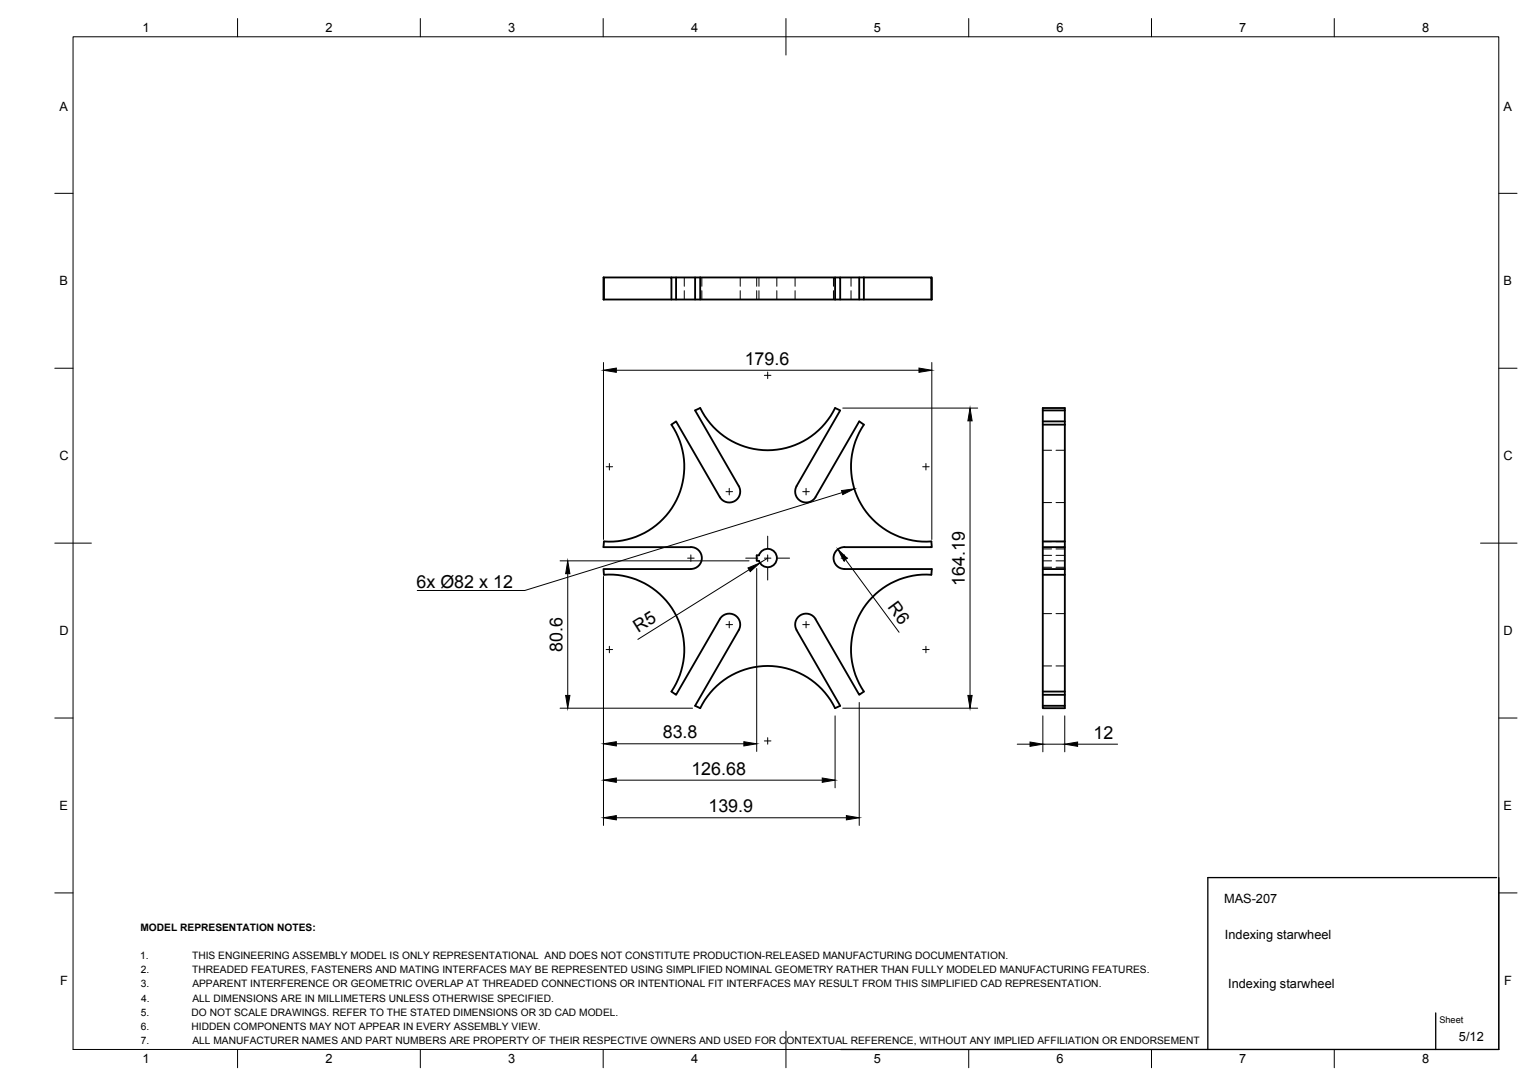
ISO-10303-21;
HEADER;
/* Generated by software containing ST-Developer
 * from STEP Tools, Inc. (www.steptools.com) 
 */

FILE_DESCRIPTION(
/* description */ ('Independent six-slot Geneva indexer. Center distance100, drive radius
50, 60degree indexing per input revolution with120degree engagement an
d240degree dwell. Native machined concave locking faces and relieved d
isk; replaceable retained drive pin; keyed output shaft. Geometry traj
ectory checks use calculated indexing positions, not a contact-dynamic
s simulation. No load or production rating assigned.'),
/* implementation_level */ '2;1');

FILE_NAME(
/* name */ 'Indexing starwheel.step',
/* time_stamp */ '2026-11-09T17:53:22-08:00',
/* author */ (''),
/* organization */ (''),
/* preprocessor_version */ 'ST-DEVELOPER v20.2',
/* originating_system */ 'Autodesk Translation Framework v15.17.0.0',
/* authorisation */ '');

FILE_SCHEMA (('AUTOMOTIVE_DESIGN { 1 0 10303 214 3 1 1 }'));
ENDSEC;

DATA;
#10=MECHANICAL_DESIGN_GEOMETRIC_PRESENTATION_REPRESENTATION('',(#103),#4149);
#81=SHAPE_REPRESENTATION_RELATIONSHIP('SRR','None',#4198,#92);
#92=ADVANCED_BREP_SHAPE_REPRESENTATION('',(#114),#4140);
#103=STYLED_ITEM('',(#4262),#114);
#114=MANIFOLD_SOLID_BREP('Body1',#2297);
#142=FACE_BOUND('',#437,.T.);
#143=FACE_BOUND('',#451,.T.);
#186=PLANE('',#2503);
#187=PLANE('',#2504);
#188=PLANE('',#2505);
#189=PLANE('',#2509);
#190=PLANE('',#2558);
#191=PLANE('',#2573);
#192=PLANE('',#2574);
#193=PLANE('',#2576);
#194=PLANE('',#2577);
#195=PLANE('',#2579);
#196=PLANE('',#2580);
#197=PLANE('',#2584);
#198=PLANE('',#2585);
#199=PLANE('',#2587);
#200=PLANE('',#2588);
#201=PLANE('',#2592);
#202=PLANE('',#2593);
#277=FACE_OUTER_BOUND('',#432,.T.);
#278=FACE_OUTER_BOUND('',#433,.T.);
#279=FACE_OUTER_BOUND('',#434,.T.);
#280=FACE_OUTER_BOUND('',#435,.T.);
#281=FACE_OUTER_BOUND('',#436,.T.);
#282=FACE_OUTER_BOUND('',#438,.T.);
#283=FACE_OUTER_BOUND('',#439,.T.);
#284=FACE_OUTER_BOUND('',#440,.T.);
#285=FACE_OUTER_BOUND('',#441,.T.);
#286=FACE_OUTER_BOUND('',#442,.T.);
#287=FACE_OUTER_BOUND('',#443,.T.);
#288=FACE_OUTER_BOUND('',#444,.T.);
#289=FACE_OUTER_BOUND('',#445,.T.);
#290=FACE_OUTER_BOUND('',#446,.T.);
#291=FACE_OUTER_BOUND('',#447,.T.);
#292=FACE_OUTER_BOUND('',#448,.T.);
#293=FACE_OUTER_BOUND('',#449,.T.);
#294=FACE_OUTER_BOUND('',#450,.T.);
#295=FACE_OUTER_BOUND('',#452,.T.);
#296=FACE_OUTER_BOUND('',#453,.T.);
#297=FACE_OUTER_BOUND('',#454,.T.);
#298=FACE_OUTER_BOUND('',#455,.T.);
#299=FACE_OUTER_BOUND('',#456,.T.);
#300=FACE_OUTER_BOUND('',#457,.T.);
#301=FACE_OUTER_BOUND('',#458,.T.);
#302=FACE_OUTER_BOUND('',#459,.T.);
#303=FACE_OUTER_BOUND('',#460,.T.);
#304=FACE_OUTER_BOUND('',#461,.T.);
#305=FACE_OUTER_BOUND('',#462,.T.);
#306=FACE_OUTER_BOUND('',#463,.T.);
#307=FACE_OUTER_BOUND('',#464,.T.);
#308=FACE_OUTER_BOUND('',#465,.T.);
#309=FACE_OUTER_BOUND('',#466,.T.);
#310=FACE_OUTER_BOUND('',#467,.T.);
#311=FACE_OUTER_BOUND('',#468,.T.);
#312=FACE_OUTER_BOUND('',#469,.T.);
#313=FACE_OUTER_BOUND('',#470,.T.);
#314=FACE_OUTER_BOUND('',#471,.T.);
#315=FACE_OUTER_BOUND('',#472,.T.);
#316=FACE_OUTER_BOUND('',#473,.T.);
#317=FACE_OUTER_BOUND('',#474,.T.);
#318=FACE_OUTER_BOUND('',#475,.T.);
#432=EDGE_LOOP('',(#1680,#1681,#1682,#1683));
#433=EDGE_LOOP('',(#1684,#1685,#1686,#1687));
#434=EDGE_LOOP('',(#1688,#1689,#1690,#1691));
#435=EDGE_LOOP('',(#1692,#1693,#1694,#1695));
#436=EDGE_LOOP('',(#1696,#1697,#1698,#1699,#1700,#1701,#1702,#1703,#1704,
#1705,#1706,#1707,#1708,#1709,#1710,#1711,#1712,#1713,#1714,#1715,#1716,
#1717,#1718,#1719,#1720,#1721,#1722,#1723,#1724,#1725,#1726,#1727,#1728,
#1729,#1730,#1731));
#437=EDGE_LOOP('',(#1732,#1733,#1734,#1735));
#438=EDGE_LOOP('',(#1736,#1737,#1738,#1739));
#439=EDGE_LOOP('',(#1740,#1741,#1742,#1743));
#440=EDGE_LOOP('',(#1744,#1745,#1746,#1747));
#441=EDGE_LOOP('',(#1748,#1749,#1750,#1751));
#442=EDGE_LOOP('',(#1752,#1753,#1754,#1755));
#443=EDGE_LOOP('',(#1756,#1757,#1758,#1759));
#444=EDGE_LOOP('',(#1760,#1761,#1762,#1763));
#445=EDGE_LOOP('',(#1764,#1765,#1766,#1767));
#446=EDGE_LOOP('',(#1768,#1769,#1770,#1771));
#447=EDGE_LOOP('',(#1772,#1773,#1774,#1775));
#448=EDGE_LOOP('',(#1776,#1777,#1778,#1779));
#449=EDGE_LOOP('',(#1780,#1781,#1782,#1783));
#450=EDGE_LOOP('',(#1784,#1785,#1786,#1787,#1788,#1789,#1790,#1791,#1792,
#1793,#1794,#1795,#1796,#1797,#1798,#1799,#1800,#1801,#1802,#1803,#1804,
#1805,#1806,#1807,#1808,#1809,#1810,#1811,#1812,#1813,#1814,#1815,#1816,
#1817,#1818,#1819));
#451=EDGE_LOOP('',(#1820,#1821,#1822,#1823));
#452=EDGE_LOOP('',(#1824,#1825,#1826,#1827));
#453=EDGE_LOOP('',(#1828,#1829,#1830,#1831));
#454=EDGE_LOOP('',(#1832,#1833,#1834,#1835));
#455=EDGE_LOOP('',(#1836,#1837,#1838,#1839));
#456=EDGE_LOOP('',(#1840,#1841,#1842,#1843));
#457=EDGE_LOOP('',(#1844,#1845,#1846,#1847));
#458=EDGE_LOOP('',(#1848,#1849,#1850,#1851));
#459=EDGE_LOOP('',(#1852,#1853,#1854,#1855));
#460=EDGE_LOOP('',(#1856,#1857,#1858,#1859));
#461=EDGE_LOOP('',(#1860,#1861,#1862,#1863));
#462=EDGE_LOOP('',(#1864,#1865,#1866,#1867));
#463=EDGE_LOOP('',(#1868,#1869,#1870,#1871));
#464=EDGE_LOOP('',(#1872,#1873,#1874,#1875));
#465=EDGE_LOOP('',(#1876,#1877,#1878,#1879));
#466=EDGE_LOOP('',(#1880,#1881,#1882,#1883));
#467=EDGE_LOOP('',(#1884,#1885,#1886,#1887));
#468=EDGE_LOOP('',(#1888,#1889,#1890,#1891));
#469=EDGE_LOOP('',(#1892,#1893,#1894,#1895));
#470=EDGE_LOOP('',(#1896,#1897,#1898,#1899));
#471=EDGE_LOOP('',(#1900,#1901,#1902,#1903));
#472=EDGE_LOOP('',(#1904,#1905,#1906,#1907));
#473=EDGE_LOOP('',(#1908,#1909,#1910,#1911));
#474=EDGE_LOOP('',(#1912,#1913,#1914,#1915));
#475=EDGE_LOOP('',(#1916,#1917,#1918,#1919));
#602=LINE('',#3655,#774);
#603=LINE('',#3657,#775);
#604=LINE('',#3659,#776);
#605=LINE('',#3660,#777);
#606=LINE('',#3664,#778);
#607=LINE('',#3666,#779);
#608=LINE('',#3668,#780);
#609=LINE('',#3669,#781);
#610=LINE('',#3671,#782);
#611=LINE('',#3672,#783);
#612=LINE('',#3683,#784);
#613=LINE('',#3687,#785);
#614=LINE('',#3695,#786);
#615=LINE('',#3699,#787);
#616=LINE('',#3707,#788);
#617=LINE('',#3711,#789);
#618=LINE('',#3719,#790);
#619=LINE('',#3723,#791);
#620=LINE('',#3731,#792);
#621=LINE('',#3735,#793);
#622=LINE('',#3743,#794);
#623=LINE('',#3747,#795);
#624=LINE('',#3751,#796);
#625=LINE('',#3753,#797);
#626=LINE('',#3757,#798);
#627=LINE('',#3759,#799);
#628=LINE('',#3763,#800);
#629=LINE('',#3765,#801);
#630=LINE('',#3769,#802);
#631=LINE('',#3771,#803);
#632=LINE('',#3775,#804);
#633=LINE('',#3777,#805);
#634=LINE('',#3781,#806);
#635=LINE('',#3784,#807);
#636=LINE('',#3787,#808);
#637=LINE('',#3792,#809);
#638=LINE('',#3795,#810);
#639=LINE('',#3799,#811);
#640=LINE('',#3803,#812);
#641=LINE('',#3807,#813);
#642=LINE('',#3811,#814);
#643=LINE('',#3815,#815);
#644=LINE('',#3818,#816);
#645=LINE('',#3822,#817);
#646=LINE('',#3825,#818);
#647=LINE('',#3829,#819);
#648=LINE('',#3832,#820);
#649=LINE('',#3836,#821);
#650=LINE('',#3839,#822);
#651=LINE('',#3843,#823);
#652=LINE('',#3848,#824);
#653=LINE('',#3851,#825);
#654=LINE('',#3853,#826);
#655=LINE('',#3855,#827);
#656=LINE('',#3857,#828);
#657=LINE('',#3859,#829);
#658=LINE('',#3862,#830);
#659=LINE('',#3863,#831);
#660=LINE('',#3865,#832);
#661=LINE('',#3868,#833);
#662=LINE('',#3869,#834);
#663=LINE('',#3871,#835);
#664=LINE('',#3876,#836);
#665=LINE('',#3877,#837);
#666=LINE('',#3879,#838);
#667=LINE('',#3882,#839);
#668=LINE('',#3883,#840);
#669=LINE('',#3885,#841);
#670=LINE('',#3890,#842);
#671=LINE('',#3892,#843);
#774=VECTOR('',#2923,10.);
#775=VECTOR('',#2924,10.);
#776=VECTOR('',#2925,10.);
#777=VECTOR('',#2926,10.);
#778=VECTOR('',#2929,10.);
#779=VECTOR('',#2930,10.);
#780=VECTOR('',#2931,10.);
#781=VECTOR('',#2932,10.);
#782=VECTOR('',#2935,10.);
#783=VECTOR('',#2936,10.);
#784=VECTOR('',#2949,10.);
#785=VECTOR('',#2952,10.);
#786=VECTOR('',#2959,10.);
#787=VECTOR('',#2962,10.);
#788=VECTOR('',#2969,10.);
#789=VECTOR('',#2972,10.);
#790=VECTOR('',#2979,10.);
#791=VECTOR('',#2982,10.);
#792=VECTOR('',#2989,10.);
#793=VECTOR('',#2992,10.);
#794=VECTOR('',#2999,10.);
#795=VECTOR('',#3002,10.);
#796=VECTOR('',#3007,10.);
#797=VECTOR('',#3008,10.);
#798=VECTOR('',#3013,10.);
#799=VECTOR('',#3014,10.);
#800=VECTOR('',#3019,10.);
#801=VECTOR('',#3020,10.);
#802=VECTOR('',#3025,10.);
#803=VECTOR('',#3026,10.);
#804=VECTOR('',#3031,10.);
#805=VECTOR('',#3032,10.);
#806=VECTOR('',#3037,10.);
#807=VECTOR('',#3040,10.);
#808=VECTOR('',#3043,10.);
#809=VECTOR('',#3050,10.);
#810=VECTOR('',#3053,10.);
#811=VECTOR('',#3058,10.);
#812=VECTOR('',#3063,10.);
#813=VECTOR('',#3068,10.);
#814=VECTOR('',#3073,10.);
#815=VECTOR('',#3076,10.);
#816=VECTOR('',#3079,10.);
#817=VECTOR('',#3082,10.);
#818=VECTOR('',#3085,10.);
#819=VECTOR('',#3088,10.);
#820=VECTOR('',#3091,10.);
#821=VECTOR('',#3094,10.);
#822=VECTOR('',#3097,10.);
#823=VECTOR('',#3100,10.);
#824=VECTOR('',#3105,10.);
#825=VECTOR('',#3108,10.);
#826=VECTOR('',#3111,10.);
#827=VECTOR('',#3114,10.);
#828=VECTOR('',#3117,10.);
#829=VECTOR('',#3120,10.);
#830=VECTOR('',#3125,10.);
#831=VECTOR('',#3126,10.);
#832=VECTOR('',#3129,10.);
#833=VECTOR('',#3134,10.);
#834=VECTOR('',#3135,10.);
#835=VECTOR('',#3138,10.);
#836=VECTOR('',#3147,10.);
#837=VECTOR('',#3148,10.);
#838=VECTOR('',#3151,10.);
#839=VECTOR('',#3156,10.);
#840=VECTOR('',#3157,10.);
#841=VECTOR('',#3160,10.);
#842=VECTOR('',#3169,10.);
#843=VECTOR('',#3172,10.);
#924=CIRCLE('',#2507,5.);
#925=CIRCLE('',#2508,5.);
#926=CIRCLE('',#2510,41.);
#927=CIRCLE('',#2511,90.);
#928=CIRCLE('',#2512,6.);
#929=CIRCLE('',#2513,90.);
#930=CIRCLE('',#2514,41.);
#931=CIRCLE('',#2515,90.);
#932=CIRCLE('',#2516,6.);
#933=CIRCLE('',#2517,90.);
#934=CIRCLE('',#2518,41.);
#935=CIRCLE('',#2519,90.);
#936=CIRCLE('',#2520,6.);
#937=CIRCLE('',#2521,90.);
#938=CIRCLE('',#2522,41.);
#939=CIRCLE('',#2523,90.);
#940=CIRCLE('',#2524,6.);
#941=CIRCLE('',#2525,90.);
#942=CIRCLE('',#2526,41.);
#943=CIRCLE('',#2527,90.);
#944=CIRCLE('',#2528,6.);
#945=CIRCLE('',#2529,90.);
#946=CIRCLE('',#2530,41.);
#947=CIRCLE('',#2531,90.);
#948=CIRCLE('',#2532,6.);
#949=CIRCLE('',#2533,90.);
#950=CIRCLE('',#2535,41.);
#951=CIRCLE('',#2537,41.);
#952=CIRCLE('',#2539,41.);
#953=CIRCLE('',#2541,41.);
#954=CIRCLE('',#2543,41.);
#955=CIRCLE('',#2545,41.);
#956=CIRCLE('',#2547,90.);
#957=CIRCLE('',#2549,90.);
#958=CIRCLE('',#2551,90.);
#959=CIRCLE('',#2553,90.);
#960=CIRCLE('',#2555,90.);
#961=CIRCLE('',#2557,90.);
#962=CIRCLE('',#2559,6.);
#963=CIRCLE('',#2560,90.);
#964=CIRCLE('',#2561,6.);
#965=CIRCLE('',#2562,90.);
#966=CIRCLE('',#2563,6.);
#967=CIRCLE('',#2564,90.);
#968=CIRCLE('',#2565,6.);
#969=CIRCLE('',#2566,90.);
#970=CIRCLE('',#2567,6.);
#971=CIRCLE('',#2568,90.);
#972=CIRCLE('',#2569,90.);
#973=CIRCLE('',#2570,6.);
#1072=VERTEX_POINT('',#3653);
#1073=VERTEX_POINT('',#3654);
#1074=VERTEX_POINT('',#3656);
#1075=VERTEX_POINT('',#3658);
#1076=VERTEX_POINT('',#3662);
#1077=VERTEX_POINT('',#3663);
#1078=VERTEX_POINT('',#3665);
#1079=VERTEX_POINT('',#3667);
#1080=VERTEX_POINT('',#3677);
#1081=VERTEX_POINT('',#3678);
#1082=VERTEX_POINT('',#3680);
#1083=VERTEX_POINT('',#3682);
#1084=VERTEX_POINT('',#3684);
#1085=VERTEX_POINT('',#3686);
#1086=VERTEX_POINT('',#3688);
#1087=VERTEX_POINT('',#3690);
#1088=VERTEX_POINT('',#3692);
#1089=VERTEX_POINT('',#3694);
#1090=VERTEX_POINT('',#3696);
#1091=VERTEX_POINT('',#3698);
#1092=VERTEX_POINT('',#3700);
#1093=VERTEX_POINT('',#3702);
#1094=VERTEX_POINT('',#3704);
#1095=VERTEX_POINT('',#3706);
#1096=VERTEX_POINT('',#3708);
#1097=VERTEX_POINT('',#3710);
#1098=VERTEX_POINT('',#3712);
#1099=VERTEX_POINT('',#3714);
#1100=VERTEX_POINT('',#3716);
#1101=VERTEX_POINT('',#3718);
#1102=VERTEX_POINT('',#3720);
#1103=VERTEX_POINT('',#3722);
#1104=VERTEX_POINT('',#3724);
#1105=VERTEX_POINT('',#3726);
#1106=VERTEX_POINT('',#3728);
#1107=VERTEX_POINT('',#3730);
#1108=VERTEX_POINT('',#3732);
#1109=VERTEX_POINT('',#3734);
#1110=VERTEX_POINT('',#3736);
#1111=VERTEX_POINT('',#3738);
#1112=VERTEX_POINT('',#3740);
#1113=VERTEX_POINT('',#3742);
#1114=VERTEX_POINT('',#3744);
#1115=VERTEX_POINT('',#3746);
#1116=VERTEX_POINT('',#3750);
#1117=VERTEX_POINT('',#3752);
#1118=VERTEX_POINT('',#3756);
#1119=VERTEX_POINT('',#3758);
#1120=VERTEX_POINT('',#3762);
#1121=VERTEX_POINT('',#3764);
#1122=VERTEX_POINT('',#3768);
#1123=VERTEX_POINT('',#3770);
#1124=VERTEX_POINT('',#3774);
#1125=VERTEX_POINT('',#3776);
#1126=VERTEX_POINT('',#3780);
#1127=VERTEX_POINT('',#3782);
#1128=VERTEX_POINT('',#3786);
#1129=VERTEX_POINT('',#3790);
#1130=VERTEX_POINT('',#3794);
#1131=VERTEX_POINT('',#3798);
#1132=VERTEX_POINT('',#3802);
#1133=VERTEX_POINT('',#3806);
#1134=VERTEX_POINT('',#3810);
#1135=VERTEX_POINT('',#3812);
#1136=VERTEX_POINT('',#3814);
#1137=VERTEX_POINT('',#3817);
#1138=VERTEX_POINT('',#3819);
#1139=VERTEX_POINT('',#3821);
#1140=VERTEX_POINT('',#3824);
#1141=VERTEX_POINT('',#3826);
#1142=VERTEX_POINT('',#3828);
#1143=VERTEX_POINT('',#3831);
#1144=VERTEX_POINT('',#3833);
#1145=VERTEX_POINT('',#3835);
#1146=VERTEX_POINT('',#3838);
#1147=VERTEX_POINT('',#3840);
#1148=VERTEX_POINT('',#3842);
#1149=VERTEX_POINT('',#3845);
#1150=VERTEX_POINT('',#3847);
#1151=VERTEX_POINT('',#3849);
#1298=EDGE_CURVE('',#1072,#1073,#602,.T.);
#1299=EDGE_CURVE('',#1074,#1072,#603,.T.);
#1300=EDGE_CURVE('',#1075,#1074,#604,.T.);
#1301=EDGE_CURVE('',#1073,#1075,#605,.T.);
#1302=EDGE_CURVE('',#1076,#1077,#606,.T.);
#1303=EDGE_CURVE('',#1078,#1076,#607,.T.);
#1304=EDGE_CURVE('',#1078,#1079,#608,.T.);
#1305=EDGE_CURVE('',#1077,#1079,#609,.T.);
#1306=EDGE_CURVE('',#1075,#1078,#610,.T.);
#1307=EDGE_CURVE('',#1079,#1074,#611,.T.);
#1308=EDGE_CURVE('',#1076,#1073,#924,.T.);
#1309=EDGE_CURVE('',#1077,#1072,#925,.T.);
#1310=EDGE_CURVE('',#1080,#1081,#926,.T.);
#1311=EDGE_CURVE('',#1081,#1082,#927,.T.);
#1312=EDGE_CURVE('',#1082,#1083,#612,.T.);
#1313=EDGE_CURVE('',#1083,#1084,#928,.T.);
#1314=EDGE_CURVE('',#1084,#1085,#613,.T.);
#1315=EDGE_CURVE('',#1085,#1086,#929,.T.);
#1316=EDGE_CURVE('',#1086,#1087,#930,.T.);
#1317=EDGE_CURVE('',#1087,#1088,#931,.T.);
#1318=EDGE_CURVE('',#1088,#1089,#614,.T.);
#1319=EDGE_CURVE('',#1089,#1090,#932,.T.);
#1320=EDGE_CURVE('',#1090,#1091,#615,.T.);
#1321=EDGE_CURVE('',#1091,#1092,#933,.T.);
#1322=EDGE_CURVE('',#1092,#1093,#934,.T.);
#1323=EDGE_CURVE('',#1093,#1094,#935,.T.);
#1324=EDGE_CURVE('',#1094,#1095,#616,.T.);
#1325=EDGE_CURVE('',#1095,#1096,#936,.T.);
#1326=EDGE_CURVE('',#1096,#1097,#617,.T.);
#1327=EDGE_CURVE('',#1097,#1098,#937,.T.);
#1328=EDGE_CURVE('',#1098,#1099,#938,.T.);
#1329=EDGE_CURVE('',#1099,#1100,#939,.T.);
#1330=EDGE_CURVE('',#1100,#1101,#618,.T.);
#1331=EDGE_CURVE('',#1101,#1102,#940,.T.);
#1332=EDGE_CURVE('',#1102,#1103,#619,.T.);
#1333=EDGE_CURVE('',#1103,#1104,#941,.T.);
#1334=EDGE_CURVE('',#1104,#1105,#942,.T.);
#1335=EDGE_CURVE('',#1105,#1106,#943,.T.);
#1336=EDGE_CURVE('',#1106,#1107,#620,.T.);
#1337=EDGE_CURVE('',#1107,#1108,#944,.T.);
#1338=EDGE_CURVE('',#1108,#1109,#621,.T.);
#1339=EDGE_CURVE('',#1109,#1110,#945,.T.);
#1340=EDGE_CURVE('',#1110,#1111,#946,.T.);
#1341=EDGE_CURVE('',#1111,#1112,#947,.T.);
#1342=EDGE_CURVE('',#1112,#1113,#622,.T.);
#1343=EDGE_CURVE('',#1113,#1114,#948,.T.);
#1344=EDGE_CURVE('',#1114,#1115,#623,.T.);
#1345=EDGE_CURVE('',#1115,#1080,#949,.T.);
#1346=EDGE_CURVE('',#1081,#1116,#624,.T.);
#1347=EDGE_CURVE('',#1117,#1080,#625,.T.);
#1348=EDGE_CURVE('',#1116,#1117,#950,.T.);
#1349=EDGE_CURVE('',#1105,#1118,#626,.T.);
#1350=EDGE_CURVE('',#1119,#1104,#627,.T.);
#1351=EDGE_CURVE('',#1118,#1119,#951,.T.);
#1352=EDGE_CURVE('',#1093,#1120,#628,.T.);
#1353=EDGE_CURVE('',#1121,#1092,#629,.T.);
#1354=EDGE_CURVE('',#1120,#1121,#952,.T.);
#1355=EDGE_CURVE('',#1099,#1122,#630,.T.);
#1356=EDGE_CURVE('',#1123,#1098,#631,.T.);
#1357=EDGE_CURVE('',#1122,#1123,#953,.T.);
#1358=EDGE_CURVE('',#1111,#1124,#632,.T.);
#1359=EDGE_CURVE('',#1125,#1110,#633,.T.);
#1360=EDGE_CURVE('',#1124,#1125,#954,.T.);
#1361=EDGE_CURVE('',#1126,#1086,#634,.T.);
#1362=EDGE_CURVE('',#1127,#1126,#955,.T.);
#1363=EDGE_CURVE('',#1087,#1127,#635,.T.);
#1364=EDGE_CURVE('',#1115,#1128,#636,.T.);
#1365=EDGE_CURVE('',#1128,#1117,#956,.T.);
#1366=EDGE_CURVE('',#1116,#1129,#957,.T.);
#1367=EDGE_CURVE('',#1129,#1082,#637,.T.);
#1368=EDGE_CURVE('',#1103,#1130,#638,.T.);
#1369=EDGE_CURVE('',#1130,#1119,#958,.T.);
#1370=EDGE_CURVE('',#1091,#1131,#639,.T.);
#1371=EDGE_CURVE('',#1131,#1121,#959,.T.);
#1372=EDGE_CURVE('',#1097,#1132,#640,.T.);
#1373=EDGE_CURVE('',#1132,#1123,#960,.T.);
#1374=EDGE_CURVE('',#1109,#1133,#641,.T.);
#1375=EDGE_CURVE('',#1133,#1125,#961,.T.);
#1376=EDGE_CURVE('',#1128,#1134,#642,.T.);
#1377=EDGE_CURVE('',#1134,#1135,#962,.T.);
#1378=EDGE_CURVE('',#1135,#1136,#643,.T.);
#1379=EDGE_CURVE('',#1124,#1136,#963,.T.);
#1380=EDGE_CURVE('',#1133,#1137,#644,.T.);
#1381=EDGE_CURVE('',#1137,#1138,#964,.T.);
#1382=EDGE_CURVE('',#1138,#1139,#645,.T.);
#1383=EDGE_CURVE('',#1118,#1139,#965,.T.);
#1384=EDGE_CURVE('',#1130,#1140,#646,.T.);
#1385=EDGE_CURVE('',#1140,#1141,#966,.T.);
#1386=EDGE_CURVE('',#1141,#1142,#647,.T.);
#1387=EDGE_CURVE('',#1122,#1142,#967,.T.);
#1388=EDGE_CURVE('',#1132,#1143,#648,.T.);
#1389=EDGE_CURVE('',#1143,#1144,#968,.T.);
#1390=EDGE_CURVE('',#1144,#1145,#649,.T.);
#1391=EDGE_CURVE('',#1120,#1145,#969,.T.);
#1392=EDGE_CURVE('',#1131,#1146,#650,.T.);
#1393=EDGE_CURVE('',#1146,#1147,#970,.T.);
#1394=EDGE_CURVE('',#1147,#1148,#651,.T.);
#1395=EDGE_CURVE('',#1127,#1148,#971,.T.);
#1396=EDGE_CURVE('',#1149,#1126,#972,.T.);
#1397=EDGE_CURVE('',#1149,#1150,#652,.T.);
#1398=EDGE_CURVE('',#1150,#1151,#973,.T.);
#1399=EDGE_CURVE('',#1151,#1129,#653,.T.);
#1400=EDGE_CURVE('',#1148,#1088,#654,.T.);
#1401=EDGE_CURVE('',#1085,#1149,#655,.T.);
#1402=EDGE_CURVE('',#1083,#1151,#656,.T.);
#1403=EDGE_CURVE('',#1084,#1150,#657,.T.);
#1404=EDGE_CURVE('',#1136,#1112,#658,.T.);
#1405=EDGE_CURVE('',#1113,#1135,#659,.T.);
#1406=EDGE_CURVE('',#1114,#1134,#660,.T.);
#1407=EDGE_CURVE('',#1139,#1106,#661,.T.);
#1408=EDGE_CURVE('',#1107,#1138,#662,.T.);
#1409=EDGE_CURVE('',#1108,#1137,#663,.T.);
#1410=EDGE_CURVE('',#1142,#1100,#664,.T.);
#1411=EDGE_CURVE('',#1101,#1141,#665,.T.);
#1412=EDGE_CURVE('',#1102,#1140,#666,.T.);
#1413=EDGE_CURVE('',#1145,#1094,#667,.T.);
#1414=EDGE_CURVE('',#1095,#1144,#668,.T.);
#1415=EDGE_CURVE('',#1096,#1143,#669,.T.);
#1416=EDGE_CURVE('',#1089,#1147,#670,.T.);
#1417=EDGE_CURVE('',#1090,#1146,#671,.T.);
#1680=ORIENTED_EDGE('',*,*,#1298,.F.);
#1681=ORIENTED_EDGE('',*,*,#1299,.F.);
#1682=ORIENTED_EDGE('',*,*,#1300,.F.);
#1683=ORIENTED_EDGE('',*,*,#1301,.F.);
#1684=ORIENTED_EDGE('',*,*,#1302,.F.);
#1685=ORIENTED_EDGE('',*,*,#1303,.F.);
#1686=ORIENTED_EDGE('',*,*,#1304,.T.);
#1687=ORIENTED_EDGE('',*,*,#1305,.F.);
#1688=ORIENTED_EDGE('',*,*,#1306,.F.);
#1689=ORIENTED_EDGE('',*,*,#1300,.T.);
#1690=ORIENTED_EDGE('',*,*,#1307,.F.);
#1691=ORIENTED_EDGE('',*,*,#1304,.F.);
#1692=ORIENTED_EDGE('',*,*,#1298,.T.);
#1693=ORIENTED_EDGE('',*,*,#1308,.F.);
#1694=ORIENTED_EDGE('',*,*,#1302,.T.);
#1695=ORIENTED_EDGE('',*,*,#1309,.T.);
#1696=ORIENTED_EDGE('',*,*,#1310,.T.);
#1697=ORIENTED_EDGE('',*,*,#1311,.T.);
#1698=ORIENTED_EDGE('',*,*,#1312,.T.);
#1699=ORIENTED_EDGE('',*,*,#1313,.T.);
#1700=ORIENTED_EDGE('',*,*,#1314,.T.);
#1701=ORIENTED_EDGE('',*,*,#1315,.T.);
#1702=ORIENTED_EDGE('',*,*,#1316,.T.);
#1703=ORIENTED_EDGE('',*,*,#1317,.T.);
#1704=ORIENTED_EDGE('',*,*,#1318,.T.);
#1705=ORIENTED_EDGE('',*,*,#1319,.T.);
#1706=ORIENTED_EDGE('',*,*,#1320,.T.);
#1707=ORIENTED_EDGE('',*,*,#1321,.T.);
#1708=ORIENTED_EDGE('',*,*,#1322,.T.);
#1709=ORIENTED_EDGE('',*,*,#1323,.T.);
#1710=ORIENTED_EDGE('',*,*,#1324,.T.);
#1711=ORIENTED_EDGE('',*,*,#1325,.T.);
#1712=ORIENTED_EDGE('',*,*,#1326,.T.);
#1713=ORIENTED_EDGE('',*,*,#1327,.T.);
#1714=ORIENTED_EDGE('',*,*,#1328,.T.);
#1715=ORIENTED_EDGE('',*,*,#1329,.T.);
#1716=ORIENTED_EDGE('',*,*,#1330,.T.);
#1717=ORIENTED_EDGE('',*,*,#1331,.T.);
#1718=ORIENTED_EDGE('',*,*,#1332,.T.);
#1719=ORIENTED_EDGE('',*,*,#1333,.T.);
#1720=ORIENTED_EDGE('',*,*,#1334,.T.);
#1721=ORIENTED_EDGE('',*,*,#1335,.T.);
#1722=ORIENTED_EDGE('',*,*,#1336,.T.);
#1723=ORIENTED_EDGE('',*,*,#1337,.T.);
#1724=ORIENTED_EDGE('',*,*,#1338,.T.);
#1725=ORIENTED_EDGE('',*,*,#1339,.T.);
#1726=ORIENTED_EDGE('',*,*,#1340,.T.);
#1727=ORIENTED_EDGE('',*,*,#1341,.T.);
#1728=ORIENTED_EDGE('',*,*,#1342,.T.);
#1729=ORIENTED_EDGE('',*,*,#1343,.T.);
#1730=ORIENTED_EDGE('',*,*,#1344,.T.);
#1731=ORIENTED_EDGE('',*,*,#1345,.T.);
#1732=ORIENTED_EDGE('',*,*,#1301,.T.);
#1733=ORIENTED_EDGE('',*,*,#1306,.T.);
#1734=ORIENTED_EDGE('',*,*,#1303,.T.);
#1735=ORIENTED_EDGE('',*,*,#1308,.T.);
#1736=ORIENTED_EDGE('',*,*,#1346,.F.);
#1737=ORIENTED_EDGE('',*,*,#1310,.F.);
#1738=ORIENTED_EDGE('',*,*,#1347,.F.);
#1739=ORIENTED_EDGE('',*,*,#1348,.F.);
#1740=ORIENTED_EDGE('',*,*,#1349,.F.);
#1741=ORIENTED_EDGE('',*,*,#1334,.F.);
#1742=ORIENTED_EDGE('',*,*,#1350,.F.);
#1743=ORIENTED_EDGE('',*,*,#1351,.F.);
#1744=ORIENTED_EDGE('',*,*,#1352,.F.);
#1745=ORIENTED_EDGE('',*,*,#1322,.F.);
#1746=ORIENTED_EDGE('',*,*,#1353,.F.);
#1747=ORIENTED_EDGE('',*,*,#1354,.F.);
#1748=ORIENTED_EDGE('',*,*,#1355,.F.);
#1749=ORIENTED_EDGE('',*,*,#1328,.F.);
#1750=ORIENTED_EDGE('',*,*,#1356,.F.);
#1751=ORIENTED_EDGE('',*,*,#1357,.F.);
#1752=ORIENTED_EDGE('',*,*,#1358,.F.);
#1753=ORIENTED_EDGE('',*,*,#1340,.F.);
#1754=ORIENTED_EDGE('',*,*,#1359,.F.);
#1755=ORIENTED_EDGE('',*,*,#1360,.F.);
#1756=ORIENTED_EDGE('',*,*,#1361,.F.);
#1757=ORIENTED_EDGE('',*,*,#1362,.F.);
#1758=ORIENTED_EDGE('',*,*,#1363,.F.);
#1759=ORIENTED_EDGE('',*,*,#1316,.F.);
#1760=ORIENTED_EDGE('',*,*,#1347,.T.);
#1761=ORIENTED_EDGE('',*,*,#1345,.F.);
#1762=ORIENTED_EDGE('',*,*,#1364,.T.);
#1763=ORIENTED_EDGE('',*,*,#1365,.T.);
#1764=ORIENTED_EDGE('',*,*,#1346,.T.);
#1765=ORIENTED_EDGE('',*,*,#1366,.T.);
#1766=ORIENTED_EDGE('',*,*,#1367,.T.);
#1767=ORIENTED_EDGE('',*,*,#1311,.F.);
#1768=ORIENTED_EDGE('',*,*,#1350,.T.);
#1769=ORIENTED_EDGE('',*,*,#1333,.F.);
#1770=ORIENTED_EDGE('',*,*,#1368,.T.);
#1771=ORIENTED_EDGE('',*,*,#1369,.T.);
#1772=ORIENTED_EDGE('',*,*,#1353,.T.);
#1773=ORIENTED_EDGE('',*,*,#1321,.F.);
#1774=ORIENTED_EDGE('',*,*,#1370,.T.);
#1775=ORIENTED_EDGE('',*,*,#1371,.T.);
#1776=ORIENTED_EDGE('',*,*,#1356,.T.);
#1777=ORIENTED_EDGE('',*,*,#1327,.F.);
#1778=ORIENTED_EDGE('',*,*,#1372,.T.);
#1779=ORIENTED_EDGE('',*,*,#1373,.T.);
#1780=ORIENTED_EDGE('',*,*,#1359,.T.);
#1781=ORIENTED_EDGE('',*,*,#1339,.F.);
#1782=ORIENTED_EDGE('',*,*,#1374,.T.);
#1783=ORIENTED_EDGE('',*,*,#1375,.T.);
#1784=ORIENTED_EDGE('',*,*,#1348,.T.);
#1785=ORIENTED_EDGE('',*,*,#1365,.F.);
#1786=ORIENTED_EDGE('',*,*,#1376,.T.);
#1787=ORIENTED_EDGE('',*,*,#1377,.T.);
#1788=ORIENTED_EDGE('',*,*,#1378,.T.);
#1789=ORIENTED_EDGE('',*,*,#1379,.F.);
#1790=ORIENTED_EDGE('',*,*,#1360,.T.);
#1791=ORIENTED_EDGE('',*,*,#1375,.F.);
#1792=ORIENTED_EDGE('',*,*,#1380,.T.);
#1793=ORIENTED_EDGE('',*,*,#1381,.T.);
#1794=ORIENTED_EDGE('',*,*,#1382,.T.);
#1795=ORIENTED_EDGE('',*,*,#1383,.F.);
#1796=ORIENTED_EDGE('',*,*,#1351,.T.);
#1797=ORIENTED_EDGE('',*,*,#1369,.F.);
#1798=ORIENTED_EDGE('',*,*,#1384,.T.);
#1799=ORIENTED_EDGE('',*,*,#1385,.T.);
#1800=ORIENTED_EDGE('',*,*,#1386,.T.);
#1801=ORIENTED_EDGE('',*,*,#1387,.F.);
#1802=ORIENTED_EDGE('',*,*,#1357,.T.);
#1803=ORIENTED_EDGE('',*,*,#1373,.F.);
#1804=ORIENTED_EDGE('',*,*,#1388,.T.);
#1805=ORIENTED_EDGE('',*,*,#1389,.T.);
#1806=ORIENTED_EDGE('',*,*,#1390,.T.);
#1807=ORIENTED_EDGE('',*,*,#1391,.F.);
#1808=ORIENTED_EDGE('',*,*,#1354,.T.);
#1809=ORIENTED_EDGE('',*,*,#1371,.F.);
#1810=ORIENTED_EDGE('',*,*,#1392,.T.);
#1811=ORIENTED_EDGE('',*,*,#1393,.T.);
#1812=ORIENTED_EDGE('',*,*,#1394,.T.);
#1813=ORIENTED_EDGE('',*,*,#1395,.F.);
#1814=ORIENTED_EDGE('',*,*,#1362,.T.);
#1815=ORIENTED_EDGE('',*,*,#1396,.F.);
#1816=ORIENTED_EDGE('',*,*,#1397,.T.);
#1817=ORIENTED_EDGE('',*,*,#1398,.T.);
#1818=ORIENTED_EDGE('',*,*,#1399,.T.);
#1819=ORIENTED_EDGE('',*,*,#1366,.F.);
#1820=ORIENTED_EDGE('',*,*,#1299,.T.);
#1821=ORIENTED_EDGE('',*,*,#1309,.F.);
#1822=ORIENTED_EDGE('',*,*,#1305,.T.);
#1823=ORIENTED_EDGE('',*,*,#1307,.T.);
#1824=ORIENTED_EDGE('',*,*,#1363,.T.);
#1825=ORIENTED_EDGE('',*,*,#1395,.T.);
#1826=ORIENTED_EDGE('',*,*,#1400,.T.);
#1827=ORIENTED_EDGE('',*,*,#1317,.F.);
#1828=ORIENTED_EDGE('',*,*,#1361,.T.);
#1829=ORIENTED_EDGE('',*,*,#1315,.F.);
#1830=ORIENTED_EDGE('',*,*,#1401,.T.);
#1831=ORIENTED_EDGE('',*,*,#1396,.T.);
#1832=ORIENTED_EDGE('',*,*,#1367,.F.);
#1833=ORIENTED_EDGE('',*,*,#1399,.F.);
#1834=ORIENTED_EDGE('',*,*,#1402,.F.);
#1835=ORIENTED_EDGE('',*,*,#1312,.F.);
#1836=ORIENTED_EDGE('',*,*,#1401,.F.);
#1837=ORIENTED_EDGE('',*,*,#1314,.F.);
#1838=ORIENTED_EDGE('',*,*,#1403,.T.);
#1839=ORIENTED_EDGE('',*,*,#1397,.F.);
#1840=ORIENTED_EDGE('',*,*,#1313,.F.);
#1841=ORIENTED_EDGE('',*,*,#1402,.T.);
#1842=ORIENTED_EDGE('',*,*,#1398,.F.);
#1843=ORIENTED_EDGE('',*,*,#1403,.F.);
#1844=ORIENTED_EDGE('',*,*,#1404,.F.);
#1845=ORIENTED_EDGE('',*,*,#1378,.F.);
#1846=ORIENTED_EDGE('',*,*,#1405,.F.);
#1847=ORIENTED_EDGE('',*,*,#1342,.F.);
#1848=ORIENTED_EDGE('',*,*,#1364,.F.);
#1849=ORIENTED_EDGE('',*,*,#1344,.F.);
#1850=ORIENTED_EDGE('',*,*,#1406,.T.);
#1851=ORIENTED_EDGE('',*,*,#1376,.F.);
#1852=ORIENTED_EDGE('',*,*,#1343,.F.);
#1853=ORIENTED_EDGE('',*,*,#1405,.T.);
#1854=ORIENTED_EDGE('',*,*,#1377,.F.);
#1855=ORIENTED_EDGE('',*,*,#1406,.F.);
#1856=ORIENTED_EDGE('',*,*,#1407,.F.);
#1857=ORIENTED_EDGE('',*,*,#1382,.F.);
#1858=ORIENTED_EDGE('',*,*,#1408,.F.);
#1859=ORIENTED_EDGE('',*,*,#1336,.F.);
#1860=ORIENTED_EDGE('',*,*,#1374,.F.);
#1861=ORIENTED_EDGE('',*,*,#1338,.F.);
#1862=ORIENTED_EDGE('',*,*,#1409,.T.);
#1863=ORIENTED_EDGE('',*,*,#1380,.F.);
#1864=ORIENTED_EDGE('',*,*,#1337,.F.);
#1865=ORIENTED_EDGE('',*,*,#1408,.T.);
#1866=ORIENTED_EDGE('',*,*,#1381,.F.);
#1867=ORIENTED_EDGE('',*,*,#1409,.F.);
#1868=ORIENTED_EDGE('',*,*,#1358,.T.);
#1869=ORIENTED_EDGE('',*,*,#1379,.T.);
#1870=ORIENTED_EDGE('',*,*,#1404,.T.);
#1871=ORIENTED_EDGE('',*,*,#1341,.F.);
#1872=ORIENTED_EDGE('',*,*,#1349,.T.);
#1873=ORIENTED_EDGE('',*,*,#1383,.T.);
#1874=ORIENTED_EDGE('',*,*,#1407,.T.);
#1875=ORIENTED_EDGE('',*,*,#1335,.F.);
#1876=ORIENTED_EDGE('',*,*,#1410,.F.);
#1877=ORIENTED_EDGE('',*,*,#1386,.F.);
#1878=ORIENTED_EDGE('',*,*,#1411,.F.);
#1879=ORIENTED_EDGE('',*,*,#1330,.F.);
#1880=ORIENTED_EDGE('',*,*,#1368,.F.);
#1881=ORIENTED_EDGE('',*,*,#1332,.F.);
#1882=ORIENTED_EDGE('',*,*,#1412,.T.);
#1883=ORIENTED_EDGE('',*,*,#1384,.F.);
#1884=ORIENTED_EDGE('',*,*,#1331,.F.);
#1885=ORIENTED_EDGE('',*,*,#1411,.T.);
#1886=ORIENTED_EDGE('',*,*,#1385,.F.);
#1887=ORIENTED_EDGE('',*,*,#1412,.F.);
#1888=ORIENTED_EDGE('',*,*,#1413,.F.);
#1889=ORIENTED_EDGE('',*,*,#1390,.F.);
#1890=ORIENTED_EDGE('',*,*,#1414,.F.);
#1891=ORIENTED_EDGE('',*,*,#1324,.F.);
#1892=ORIENTED_EDGE('',*,*,#1372,.F.);
#1893=ORIENTED_EDGE('',*,*,#1326,.F.);
#1894=ORIENTED_EDGE('',*,*,#1415,.T.);
#1895=ORIENTED_EDGE('',*,*,#1388,.F.);
#1896=ORIENTED_EDGE('',*,*,#1325,.F.);
#1897=ORIENTED_EDGE('',*,*,#1414,.T.);
#1898=ORIENTED_EDGE('',*,*,#1389,.F.);
#1899=ORIENTED_EDGE('',*,*,#1415,.F.);
#1900=ORIENTED_EDGE('',*,*,#1355,.T.);
#1901=ORIENTED_EDGE('',*,*,#1387,.T.);
#1902=ORIENTED_EDGE('',*,*,#1410,.T.);
#1903=ORIENTED_EDGE('',*,*,#1329,.F.);
#1904=ORIENTED_EDGE('',*,*,#1352,.T.);
#1905=ORIENTED_EDGE('',*,*,#1391,.T.);
#1906=ORIENTED_EDGE('',*,*,#1413,.T.);
#1907=ORIENTED_EDGE('',*,*,#1323,.F.);
#1908=ORIENTED_EDGE('',*,*,#1400,.F.);
#1909=ORIENTED_EDGE('',*,*,#1394,.F.);
#1910=ORIENTED_EDGE('',*,*,#1416,.F.);
#1911=ORIENTED_EDGE('',*,*,#1318,.F.);
#1912=ORIENTED_EDGE('',*,*,#1370,.F.);
#1913=ORIENTED_EDGE('',*,*,#1320,.F.);
#1914=ORIENTED_EDGE('',*,*,#1417,.T.);
#1915=ORIENTED_EDGE('',*,*,#1392,.F.);
#1916=ORIENTED_EDGE('',*,*,#1319,.F.);
#1917=ORIENTED_EDGE('',*,*,#1416,.T.);
#1918=ORIENTED_EDGE('',*,*,#1393,.F.);
#1919=ORIENTED_EDGE('',*,*,#1417,.F.);
#2114=CYLINDRICAL_SURFACE('',#2506,5.);
#2115=CYLINDRICAL_SURFACE('',#2534,41.);
#2116=CYLINDRICAL_SURFACE('',#2536,41.);
#2117=CYLINDRICAL_SURFACE('',#2538,41.);
#2118=CYLINDRICAL_SURFACE('',#2540,41.);
#2119=CYLINDRICAL_SURFACE('',#2542,41.);
#2120=CYLINDRICAL_SURFACE('',#2544,41.);
#2121=CYLINDRICAL_SURFACE('',#2546,90.);
#2122=CYLINDRICAL_SURFACE('',#2548,90.);
#2123=CYLINDRICAL_SURFACE('',#2550,90.);
#2124=CYLINDRICAL_SURFACE('',#2552,90.);
#2125=CYLINDRICAL_SURFACE('',#2554,90.);
#2126=CYLINDRICAL_SURFACE('',#2556,90.);
#2127=CYLINDRICAL_SURFACE('',#2571,90.);
#2128=CYLINDRICAL_SURFACE('',#2572,90.);
#2129=CYLINDRICAL_SURFACE('',#2575,6.);
#2130=CYLINDRICAL_SURFACE('',#2578,6.);
#2131=CYLINDRICAL_SURFACE('',#2581,6.);
#2132=CYLINDRICAL_SURFACE('',#2582,90.);
#2133=CYLINDRICAL_SURFACE('',#2583,90.);
#2134=CYLINDRICAL_SURFACE('',#2586,6.);
#2135=CYLINDRICAL_SURFACE('',#2589,6.);
#2136=CYLINDRICAL_SURFACE('',#2590,90.);
#2137=CYLINDRICAL_SURFACE('',#2591,90.);
#2138=CYLINDRICAL_SURFACE('',#2594,6.);
#2198=ADVANCED_FACE('',(#277),#186,.F.);
#2199=ADVANCED_FACE('',(#278),#187,.F.);
#2200=ADVANCED_FACE('',(#279),#188,.F.);
#2201=ADVANCED_FACE('',(#280),#2114,.F.);
#2202=ADVANCED_FACE('',(#281,#142),#189,.T.);
#2203=ADVANCED_FACE('',(#282),#2115,.F.);
#2204=ADVANCED_FACE('',(#283),#2116,.F.);
#2205=ADVANCED_FACE('',(#284),#2117,.F.);
#2206=ADVANCED_FACE('',(#285),#2118,.F.);
#2207=ADVANCED_FACE('',(#286),#2119,.F.);
#2208=ADVANCED_FACE('',(#287),#2120,.F.);
#2209=ADVANCED_FACE('',(#288),#2121,.T.);
#2210=ADVANCED_FACE('',(#289),#2122,.T.);
#2211=ADVANCED_FACE('',(#290),#2123,.T.);
#2212=ADVANCED_FACE('',(#291),#2124,.T.);
#2213=ADVANCED_FACE('',(#292),#2125,.T.);
#2214=ADVANCED_FACE('',(#293),#2126,.T.);
#2215=ADVANCED_FACE('',(#294,#143),#190,.F.);
#2216=ADVANCED_FACE('',(#295),#2127,.T.);
#2217=ADVANCED_FACE('',(#296),#2128,.T.);
#2218=ADVANCED_FACE('',(#297),#191,.F.);
#2219=ADVANCED_FACE('',(#298),#192,.F.);
#2220=ADVANCED_FACE('',(#299),#2129,.F.);
#2221=ADVANCED_FACE('',(#300),#193,.F.);
#2222=ADVANCED_FACE('',(#301),#194,.F.);
#2223=ADVANCED_FACE('',(#302),#2130,.F.);
#2224=ADVANCED_FACE('',(#303),#195,.F.);
#2225=ADVANCED_FACE('',(#304),#196,.F.);
#2226=ADVANCED_FACE('',(#305),#2131,.F.);
#2227=ADVANCED_FACE('',(#306),#2132,.T.);
#2228=ADVANCED_FACE('',(#307),#2133,.T.);
#2229=ADVANCED_FACE('',(#308),#197,.F.);
#2230=ADVANCED_FACE('',(#309),#198,.F.);
#2231=ADVANCED_FACE('',(#310),#2134,.F.);
#2232=ADVANCED_FACE('',(#311),#199,.F.);
#2233=ADVANCED_FACE('',(#312),#200,.F.);
#2234=ADVANCED_FACE('',(#313),#2135,.F.);
#2235=ADVANCED_FACE('',(#314),#2136,.T.);
#2236=ADVANCED_FACE('',(#315),#2137,.T.);
#2237=ADVANCED_FACE('',(#316),#201,.F.);
#2238=ADVANCED_FACE('',(#317),#202,.F.);
#2239=ADVANCED_FACE('',(#318),#2138,.F.);
#2297=CLOSED_SHELL('',(#2198,#2199,#2200,#2201,#2202,#2203,#2204,#2205,
#2206,#2207,#2208,#2209,#2210,#2211,#2212,#2213,#2214,#2215,#2216,#2217,
#2218,#2219,#2220,#2221,#2222,#2223,#2224,#2225,#2226,#2227,#2228,#2229,
#2230,#2231,#2232,#2233,#2234,#2235,#2236,#2237,#2238,#2239));
#2502=AXIS2_PLACEMENT_3D('',#3651,#2919,#2920);
#2503=AXIS2_PLACEMENT_3D('',#3652,#2921,#2922);
#2504=AXIS2_PLACEMENT_3D('',#3661,#2927,#2928);
#2505=AXIS2_PLACEMENT_3D('',#3670,#2933,#2934);
#2506=AXIS2_PLACEMENT_3D('',#3673,#2937,#2938);
#2507=AXIS2_PLACEMENT_3D('',#3674,#2939,#2940);
#2508=AXIS2_PLACEMENT_3D('',#3675,#2941,#2942);
#2509=AXIS2_PLACEMENT_3D('',#3676,#2943,#2944);
#2510=AXIS2_PLACEMENT_3D('',#3679,#2945,#2946);
#2511=AXIS2_PLACEMENT_3D('',#3681,#2947,#2948);
#2512=AXIS2_PLACEMENT_3D('',#3685,#2950,#2951);
#2513=AXIS2_PLACEMENT_3D('',#3689,#2953,#2954);
#2514=AXIS2_PLACEMENT_3D('',#3691,#2955,#2956);
#2515=AXIS2_PLACEMENT_3D('',#3693,#2957,#2958);
#2516=AXIS2_PLACEMENT_3D('',#3697,#2960,#2961);
#2517=AXIS2_PLACEMENT_3D('',#3701,#2963,#2964);
#2518=AXIS2_PLACEMENT_3D('',#3703,#2965,#2966);
#2519=AXIS2_PLACEMENT_3D('',#3705,#2967,#2968);
#2520=AXIS2_PLACEMENT_3D('',#3709,#2970,#2971);
#2521=AXIS2_PLACEMENT_3D('',#3713,#2973,#2974);
#2522=AXIS2_PLACEMENT_3D('',#3715,#2975,#2976);
#2523=AXIS2_PLACEMENT_3D('',#3717,#2977,#2978);
#2524=AXIS2_PLACEMENT_3D('',#3721,#2980,#2981);
#2525=AXIS2_PLACEMENT_3D('',#3725,#2983,#2984);
#2526=AXIS2_PLACEMENT_3D('',#3727,#2985,#2986);
#2527=AXIS2_PLACEMENT_3D('',#3729,#2987,#2988);
#2528=AXIS2_PLACEMENT_3D('',#3733,#2990,#2991);
#2529=AXIS2_PLACEMENT_3D('',#3737,#2993,#2994);
#2530=AXIS2_PLACEMENT_3D('',#3739,#2995,#2996);
#2531=AXIS2_PLACEMENT_3D('',#3741,#2997,#2998);
#2532=AXIS2_PLACEMENT_3D('',#3745,#3000,#3001);
#2533=AXIS2_PLACEMENT_3D('',#3748,#3003,#3004);
#2534=AXIS2_PLACEMENT_3D('',#3749,#3005,#3006);
#2535=AXIS2_PLACEMENT_3D('',#3754,#3009,#3010);
#2536=AXIS2_PLACEMENT_3D('',#3755,#3011,#3012);
#2537=AXIS2_PLACEMENT_3D('',#3760,#3015,#3016);
#2538=AXIS2_PLACEMENT_3D('',#3761,#3017,#3018);
#2539=AXIS2_PLACEMENT_3D('',#3766,#3021,#3022);
#2540=AXIS2_PLACEMENT_3D('',#3767,#3023,#3024);
#2541=AXIS2_PLACEMENT_3D('',#3772,#3027,#3028);
#2542=AXIS2_PLACEMENT_3D('',#3773,#3029,#3030);
#2543=AXIS2_PLACEMENT_3D('',#3778,#3033,#3034);
#2544=AXIS2_PLACEMENT_3D('',#3779,#3035,#3036);
#2545=AXIS2_PLACEMENT_3D('',#3783,#3038,#3039);
#2546=AXIS2_PLACEMENT_3D('',#3785,#3041,#3042);
#2547=AXIS2_PLACEMENT_3D('',#3788,#3044,#3045);
#2548=AXIS2_PLACEMENT_3D('',#3789,#3046,#3047);
#2549=AXIS2_PLACEMENT_3D('',#3791,#3048,#3049);
#2550=AXIS2_PLACEMENT_3D('',#3793,#3051,#3052);
#2551=AXIS2_PLACEMENT_3D('',#3796,#3054,#3055);
#2552=AXIS2_PLACEMENT_3D('',#3797,#3056,#3057);
#2553=AXIS2_PLACEMENT_3D('',#3800,#3059,#3060);
#2554=AXIS2_PLACEMENT_3D('',#3801,#3061,#3062);
#2555=AXIS2_PLACEMENT_3D('',#3804,#3064,#3065);
#2556=AXIS2_PLACEMENT_3D('',#3805,#3066,#3067);
#2557=AXIS2_PLACEMENT_3D('',#3808,#3069,#3070);
#2558=AXIS2_PLACEMENT_3D('',#3809,#3071,#3072);
#2559=AXIS2_PLACEMENT_3D('',#3813,#3074,#3075);
#2560=AXIS2_PLACEMENT_3D('',#3816,#3077,#3078);
#2561=AXIS2_PLACEMENT_3D('',#3820,#3080,#3081);
#2562=AXIS2_PLACEMENT_3D('',#3823,#3083,#3084);
#2563=AXIS2_PLACEMENT_3D('',#3827,#3086,#3087);
#2564=AXIS2_PLACEMENT_3D('',#3830,#3089,#3090);
#2565=AXIS2_PLACEMENT_3D('',#3834,#3092,#3093);
#2566=AXIS2_PLACEMENT_3D('',#3837,#3095,#3096);
#2567=AXIS2_PLACEMENT_3D('',#3841,#3098,#3099);
#2568=AXIS2_PLACEMENT_3D('',#3844,#3101,#3102);
#2569=AXIS2_PLACEMENT_3D('',#3846,#3103,#3104);
#2570=AXIS2_PLACEMENT_3D('',#3850,#3106,#3107);
#2571=AXIS2_PLACEMENT_3D('',#3852,#3109,#3110);
#2572=AXIS2_PLACEMENT_3D('',#3854,#3112,#3113);
#2573=AXIS2_PLACEMENT_3D('',#3856,#3115,#3116);
#2574=AXIS2_PLACEMENT_3D('',#3858,#3118,#3119);
#2575=AXIS2_PLACEMENT_3D('',#3860,#3121,#3122);
#2576=AXIS2_PLACEMENT_3D('',#3861,#3123,#3124);
#2577=AXIS2_PLACEMENT_3D('',#3864,#3127,#3128);
#2578=AXIS2_PLACEMENT_3D('',#3866,#3130,#3131);
#2579=AXIS2_PLACEMENT_3D('',#3867,#3132,#3133);
#2580=AXIS2_PLACEMENT_3D('',#3870,#3136,#3137);
#2581=AXIS2_PLACEMENT_3D('',#3872,#3139,#3140);
#2582=AXIS2_PLACEMENT_3D('',#3873,#3141,#3142);
#2583=AXIS2_PLACEMENT_3D('',#3874,#3143,#3144);
#2584=AXIS2_PLACEMENT_3D('',#3875,#3145,#3146);
#2585=AXIS2_PLACEMENT_3D('',#3878,#3149,#3150);
#2586=AXIS2_PLACEMENT_3D('',#3880,#3152,#3153);
#2587=AXIS2_PLACEMENT_3D('',#3881,#3154,#3155);
#2588=AXIS2_PLACEMENT_3D('',#3884,#3158,#3159);
#2589=AXIS2_PLACEMENT_3D('',#3886,#3161,#3162);
#2590=AXIS2_PLACEMENT_3D('',#3887,#3163,#3164);
#2591=AXIS2_PLACEMENT_3D('',#3888,#3165,#3166);
#2592=AXIS2_PLACEMENT_3D('',#3889,#3167,#3168);
#2593=AXIS2_PLACEMENT_3D('',#3891,#3170,#3171);
#2594=AXIS2_PLACEMENT_3D('',#3893,#3173,#3174);
#2919=DIRECTION('axis',(0.,0.,1.));
#2920=DIRECTION('refdir',(1.,0.,0.));
#2921=DIRECTION('center_axis',(0.,1.,0.));
#2922=DIRECTION('ref_axis',(1.,0.,0.));
#2923=DIRECTION('',(0.,0.,1.));
#2924=DIRECTION('',(-1.,0.,0.));
#2925=DIRECTION('',(0.,0.,-1.));
#2926=DIRECTION('',(1.,0.,0.));
#2927=DIRECTION('center_axis',(0.,-1.,0.));
#2928=DIRECTION('ref_axis',(-1.,0.,0.));
#2929=DIRECTION('',(0.,0.,-1.));
#2930=DIRECTION('',(-1.,0.,0.));
#2931=DIRECTION('',(0.,0.,-1.));
#2932=DIRECTION('',(1.,0.,0.));
#2933=DIRECTION('center_axis',(1.,0.,0.));
#2934=DIRECTION('ref_axis',(0.,-1.,0.));
#2935=DIRECTION('',(0.,-1.,0.));
#2936=DIRECTION('',(0.,1.,0.));
#2937=DIRECTION('center_axis',(0.,0.,1.));
#2938=DIRECTION('ref_axis',(-1.,1.22464679914735E-16,0.));
#2939=DIRECTION('center_axis',(0.,0.,-1.));
#2940=DIRECTION('ref_axis',(1.,0.,0.));
#2941=DIRECTION('center_axis',(0.,0.,-1.));
#2942=DIRECTION('ref_axis',(1.,0.,0.));
#2943=DIRECTION('center_axis',(0.,0.,1.));
#2944=DIRECTION('ref_axis',(1.,0.,0.));
#2945=DIRECTION('center_axis',(0.,0.,-1.));
#2946=DIRECTION('ref_axis',(1.,0.,0.));
#2947=DIRECTION('center_axis',(0.,0.,1.));
#2948=DIRECTION('ref_axis',(1.,0.,0.));
#2949=DIRECTION('',(-0.5,0.866025403784439,0.));
#2950=DIRECTION('center_axis',(0.,0.,-1.));
#2951=DIRECTION('ref_axis',(0.866025403784439,0.5,0.));
#2952=DIRECTION('',(0.5,-0.866025403784439,0.));
#2953=DIRECTION('center_axis',(0.,0.,1.));
#2954=DIRECTION('ref_axis',(1.,0.,0.));
#2955=DIRECTION('center_axis',(0.,0.,-1.));
#2956=DIRECTION('ref_axis',(1.,0.,0.));
#2957=DIRECTION('center_axis',(0.,0.,1.));
#2958=DIRECTION('ref_axis',(1.,0.,0.));
#2959=DIRECTION('',(-1.,0.,0.));
#2960=DIRECTION('center_axis',(0.,0.,-1.));
#2961=DIRECTION('ref_axis',(0.,1.,0.));
#2962=DIRECTION('',(1.,0.,0.));
#2963=DIRECTION('center_axis',(0.,0.,1.));
#2964=DIRECTION('ref_axis',(1.,0.,0.));
#2965=DIRECTION('center_axis',(0.,0.,-1.));
#2966=DIRECTION('ref_axis',(1.,0.,0.));
#2967=DIRECTION('center_axis',(0.,0.,1.));
#2968=DIRECTION('ref_axis',(1.,0.,0.));
#2969=DIRECTION('',(-0.5,-0.866025403784439,0.));
#2970=DIRECTION('center_axis',(0.,0.,-1.));
#2971=DIRECTION('ref_axis',(-0.866025403784439,0.5,0.));
#2972=DIRECTION('',(0.5,0.866025403784439,0.));
#2973=DIRECTION('center_axis',(0.,0.,1.));
#2974=DIRECTION('ref_axis',(1.,0.,0.));
#2975=DIRECTION('center_axis',(0.,0.,-1.));
#2976=DIRECTION('ref_axis',(1.,0.,0.));
#2977=DIRECTION('center_axis',(0.,0.,1.));
#2978=DIRECTION('ref_axis',(1.,0.,0.));
#2979=DIRECTION('',(0.5,-0.866025403784439,0.));
#2980=DIRECTION('center_axis',(0.,0.,-1.));
#2981=DIRECTION('ref_axis',(-0.866025403784439,-0.5,0.));
#2982=DIRECTION('',(-0.5,0.866025403784439,0.));
#2983=DIRECTION('center_axis',(0.,0.,1.));
#2984=DIRECTION('ref_axis',(1.,0.,0.));
#2985=DIRECTION('center_axis',(0.,0.,-1.));
#2986=DIRECTION('ref_axis',(1.,0.,0.));
#2987=DIRECTION('center_axis',(0.,0.,1.));
#2988=DIRECTION('ref_axis',(1.,0.,0.));
#2989=DIRECTION('',(1.,-1.14850657719844E-16,0.));
#2990=DIRECTION('center_axis',(0.,0.,-1.));
#2991=DIRECTION('ref_axis',(0.,-1.,0.));
#2992=DIRECTION('',(-1.,1.14850657719844E-16,0.));
#2993=DIRECTION('center_axis',(0.,0.,1.));
#2994=DIRECTION('ref_axis',(1.,0.,0.));
#2995=DIRECTION('center_axis',(0.,0.,-1.));
#2996=DIRECTION('ref_axis',(1.,0.,0.));
#2997=DIRECTION('center_axis',(0.,0.,1.));
#2998=DIRECTION('ref_axis',(1.,0.,0.));
#2999=DIRECTION('',(0.5,0.866025403784438,0.));
#3000=DIRECTION('center_axis',(0.,0.,-1.));
#3001=DIRECTION('ref_axis',(0.866025403784438,-0.5,0.));
#3002=DIRECTION('',(-0.5,-0.866025403784439,0.));
#3003=DIRECTION('center_axis',(0.,0.,1.));
#3004=DIRECTION('ref_axis',(1.,0.,0.));
#3005=DIRECTION('center_axis',(0.,0.,-1.));
#3006=DIRECTION('ref_axis',(1.,0.,0.));
#3007=DIRECTION('',(0.,0.,-1.));
#3008=DIRECTION('',(0.,0.,1.));
#3009=DIRECTION('center_axis',(0.,0.,1.));
#3010=DIRECTION('ref_axis',(1.,0.,0.));
#3011=DIRECTION('center_axis',(0.,0.,-1.));
#3012=DIRECTION('ref_axis',(1.,0.,0.));
#3013=DIRECTION('',(0.,0.,-1.));
#3014=DIRECTION('',(0.,0.,1.));
#3015=DIRECTION('center_axis',(0.,0.,1.));
#3016=DIRECTION('ref_axis',(1.,0.,0.));
#3017=DIRECTION('center_axis',(0.,0.,-1.));
#3018=DIRECTION('ref_axis',(-0.866025403784439,-0.499999999999999,0.));
#3019=DIRECTION('',(0.,0.,-1.));
#3020=DIRECTION('',(0.,0.,1.));
#3021=DIRECTION('center_axis',(0.,0.,1.));
#3022=DIRECTION('ref_axis',(1.,0.,0.));
#3023=DIRECTION('center_axis',(0.,0.,-1.));
#3024=DIRECTION('ref_axis',(1.,0.,0.));
#3025=DIRECTION('',(0.,0.,-1.));
#3026=DIRECTION('',(0.,0.,1.));
#3027=DIRECTION('center_axis',(0.,0.,1.));
#3028=DIRECTION('ref_axis',(1.,0.,0.));
#3029=DIRECTION('center_axis',(0.,0.,-1.));
#3030=DIRECTION('ref_axis',(1.,0.,0.));
#3031=DIRECTION('',(0.,0.,-1.));
#3032=DIRECTION('',(0.,0.,1.));
#3033=DIRECTION('center_axis',(0.,0.,1.));
#3034=DIRECTION('ref_axis',(1.,0.,0.));
#3035=DIRECTION('center_axis',(0.,0.,-1.));
#3036=DIRECTION('ref_axis',(-0.866025403784439,0.5,0.));
#3037=DIRECTION('',(0.,0.,1.));
#3038=DIRECTION('center_axis',(0.,0.,1.));
#3039=DIRECTION('ref_axis',(1.,0.,0.));
#3040=DIRECTION('',(0.,0.,-1.));
#3041=DIRECTION('center_axis',(0.,0.,1.));
#3042=DIRECTION('ref_axis',(1.,0.,0.));
#3043=DIRECTION('',(0.,0.,-1.));
#3044=DIRECTION('center_axis',(0.,0.,1.));
#3045=DIRECTION('ref_axis',(1.,0.,0.));
#3046=DIRECTION('center_axis',(0.,0.,1.));
#3047=DIRECTION('ref_axis',(1.,0.,0.));
#3048=DIRECTION('center_axis',(0.,0.,1.));
#3049=DIRECTION('ref_axis',(1.,0.,0.));
#3050=DIRECTION('',(0.,0.,1.));
#3051=DIRECTION('center_axis',(0.,0.,1.));
#3052=DIRECTION('ref_axis',(1.,0.,0.));
#3053=DIRECTION('',(0.,0.,-1.));
#3054=DIRECTION('center_axis',(0.,0.,1.));
#3055=DIRECTION('ref_axis',(1.,0.,0.));
#3056=DIRECTION('center_axis',(0.,0.,1.));
#3057=DIRECTION('ref_axis',(1.,0.,0.));
#3058=DIRECTION('',(0.,0.,-1.));
#3059=DIRECTION('center_axis',(0.,0.,1.));
#3060=DIRECTION('ref_axis',(1.,0.,0.));
#3061=DIRECTION('center_axis',(0.,0.,1.));
#3062=DIRECTION('ref_axis',(1.,0.,0.));
#3063=DIRECTION('',(0.,0.,-1.));
#3064=DIRECTION('center_axis',(0.,0.,1.));
#3065=DIRECTION('ref_axis',(1.,0.,0.));
#3066=DIRECTION('center_axis',(0.,0.,1.));
#3067=DIRECTION('ref_axis',(1.,0.,0.));
#3068=DIRECTION('',(0.,0.,-1.));
#3069=DIRECTION('center_axis',(0.,0.,1.));
#3070=DIRECTION('ref_axis',(1.,0.,0.));
#3071=DIRECTION('center_axis',(0.,0.,1.));
#3072=DIRECTION('ref_axis',(1.,0.,0.));
#3073=DIRECTION('',(0.5,0.866025403784439,0.));
#3074=DIRECTION('center_axis',(0.,0.,1.));
#3075=DIRECTION('ref_axis',(0.866025403784438,-0.5,0.));
#3076=DIRECTION('',(-0.5,-0.866025403784438,0.));
#3077=DIRECTION('center_axis',(0.,0.,1.));
#3078=DIRECTION('ref_axis',(1.,0.,0.));
#3079=DIRECTION('',(1.,-1.14850657719844E-16,0.));
#3080=DIRECTION('center_axis',(0.,0.,1.));
#3081=DIRECTION('ref_axis',(0.,-1.,0.));
#3082=DIRECTION('',(-1.,1.14850657719844E-16,0.));
#3083=DIRECTION('center_axis',(0.,0.,1.));
#3084=DIRECTION('ref_axis',(1.,0.,0.));
#3085=DIRECTION('',(0.5,-0.866025403784439,0.));
#3086=DIRECTION('center_axis',(0.,0.,1.));
#3087=DIRECTION('ref_axis',(-0.866025403784439,-0.5,0.));
#3088=DIRECTION('',(-0.5,0.866025403784439,0.));
#3089=DIRECTION('center_axis',(0.,0.,1.));
#3090=DIRECTION('ref_axis',(1.,0.,0.));
#3091=DIRECTION('',(-0.5,-0.866025403784439,0.));
#3092=DIRECTION('center_axis',(0.,0.,1.));
#3093=DIRECTION('ref_axis',(-0.866025403784439,0.5,0.));
#3094=DIRECTION('',(0.5,0.866025403784439,0.));
#3095=DIRECTION('center_axis',(0.,0.,1.));
#3096=DIRECTION('ref_axis',(1.,0.,0.));
#3097=DIRECTION('',(-1.,0.,0.));
#3098=DIRECTION('center_axis',(0.,0.,1.));
#3099=DIRECTION('ref_axis',(0.,1.,0.));
#3100=DIRECTION('',(1.,0.,0.));
#3101=DIRECTION('center_axis',(0.,0.,1.));
#3102=DIRECTION('ref_axis',(1.,0.,0.));
#3103=DIRECTION('center_axis',(0.,0.,1.));
#3104=DIRECTION('ref_axis',(1.,0.,0.));
#3105=DIRECTION('',(-0.5,0.866025403784439,0.));
#3106=DIRECTION('center_axis',(0.,0.,1.));
#3107=DIRECTION('ref_axis',(0.866025403784439,0.5,0.));
#3108=DIRECTION('',(0.5,-0.866025403784439,0.));
#3109=DIRECTION('center_axis',(0.,0.,1.));
#3110=DIRECTION('ref_axis',(1.,0.,0.));
#3111=DIRECTION('',(0.,0.,1.));
#3112=DIRECTION('center_axis',(0.,0.,1.));
#3113=DIRECTION('ref_axis',(1.,0.,0.));
#3114=DIRECTION('',(0.,0.,-1.));
#3115=DIRECTION('center_axis',(-0.866025403784439,-0.5,0.));
#3116=DIRECTION('ref_axis',(-0.5,0.866025403784439,0.));
#3117=DIRECTION('',(0.,0.,-1.));
#3118=DIRECTION('center_axis',(0.866025403784439,0.5,0.));
#3119=DIRECTION('ref_axis',(0.5,-0.866025403784439,0.));
#3120=DIRECTION('',(0.,0.,-1.));
#3121=DIRECTION('center_axis',(0.,0.,-1.));
#3122=DIRECTION('ref_axis',(0.866025403784439,0.5,0.));
#3123=DIRECTION('center_axis',(-0.866025403784438,0.5,0.));
#3124=DIRECTION('ref_axis',(0.5,0.866025403784438,0.));
#3125=DIRECTION('',(0.,0.,1.));
#3126=DIRECTION('',(0.,0.,-1.));
#3127=DIRECTION('center_axis',(0.866025403784439,-0.5,0.));
#3128=DIRECTION('ref_axis',(-0.5,-0.866025403784439,0.));
#3129=DIRECTION('',(0.,0.,-1.));
#3130=DIRECTION('center_axis',(0.,0.,-1.));
#3131=DIRECTION('ref_axis',(0.866025403784438,-0.5,0.));
#3132=DIRECTION('center_axis',(1.14850657719844E-16,1.,0.));
#3133=DIRECTION('ref_axis',(1.,-1.14850657719844E-16,0.));
#3134=DIRECTION('',(0.,0.,1.));
#3135=DIRECTION('',(0.,0.,-1.));
#3136=DIRECTION('center_axis',(-1.14850657719844E-16,-1.,0.));
#3137=DIRECTION('ref_axis',(-1.,1.14850657719844E-16,0.));
#3138=DIRECTION('',(0.,0.,-1.));
#3139=DIRECTION('center_axis',(0.,0.,-1.));
#3140=DIRECTION('ref_axis',(0.,-1.,0.));
#3141=DIRECTION('center_axis',(0.,0.,1.));
#3142=DIRECTION('ref_axis',(1.,0.,0.));
#3143=DIRECTION('center_axis',(0.,0.,1.));
#3144=DIRECTION('ref_axis',(1.,0.,0.));
#3145=DIRECTION('center_axis',(0.866025403784439,0.5,0.));
#3146=DIRECTION('ref_axis',(0.5,-0.866025403784439,0.));
#3147=DIRECTION('',(0.,0.,1.));
#3148=DIRECTION('',(0.,0.,-1.));
#3149=DIRECTION('center_axis',(-0.866025403784439,-0.5,0.));
#3150=DIRECTION('ref_axis',(-0.5,0.866025403784439,0.));
#3151=DIRECTION('',(0.,0.,-1.));
#3152=DIRECTION('center_axis',(0.,0.,-1.));
#3153=DIRECTION('ref_axis',(-0.866025403784439,-0.5,0.));
#3154=DIRECTION('center_axis',(0.866025403784439,-0.5,0.));
#3155=DIRECTION('ref_axis',(-0.5,-0.866025403784439,0.));
#3156=DIRECTION('',(0.,0.,1.));
#3157=DIRECTION('',(0.,0.,-1.));
#3158=DIRECTION('center_axis',(-0.866025403784439,0.5,0.));
#3159=DIRECTION('ref_axis',(0.5,0.866025403784439,0.));
#3160=DIRECTION('',(0.,0.,-1.));
#3161=DIRECTION('center_axis',(0.,0.,-1.));
#3162=DIRECTION('ref_axis',(-0.866025403784439,0.5,0.));
#3163=DIRECTION('center_axis',(0.,0.,1.));
#3164=DIRECTION('ref_axis',(1.,0.,0.));
#3165=DIRECTION('center_axis',(0.,0.,1.));
#3166=DIRECTION('ref_axis',(1.,0.,0.));
#3167=DIRECTION('center_axis',(0.,-1.,0.));
#3168=DIRECTION('ref_axis',(-1.,0.,0.));
#3169=DIRECTION('',(0.,0.,-1.));
#3170=DIRECTION('center_axis',(0.,1.,0.));
#3171=DIRECTION('ref_axis',(1.,0.,0.));
#3172=DIRECTION('',(0.,0.,-1.));
#3173=DIRECTION('center_axis',(0.,0.,-1.));
#3174=DIRECTION('ref_axis',(0.,1.,0.));
#3651=CARTESIAN_POINT('',(0.,0.,0.));
#3652=CARTESIAN_POINT('Origin',(3.,1.5,12.));
#3653=CARTESIAN_POINT('',(4.76969600708473,1.5,0.));
#3654=CARTESIAN_POINT('',(4.76969600708473,1.5,12.));
#3655=CARTESIAN_POINT('',(4.76969600708473,1.5,0.));
#3656=CARTESIAN_POINT('',(6.,1.5,0.));
#3657=CARTESIAN_POINT('',(1.5,1.5,0.));
#3658=CARTESIAN_POINT('',(6.,1.5,12.));
#3659=CARTESIAN_POINT('',(6.,1.5,12.));
#3660=CARTESIAN_POINT('',(1.5,1.5,12.));
#3661=CARTESIAN_POINT('Origin',(6.,-1.5,12.));
#3662=CARTESIAN_POINT('',(4.76969600708473,-1.5,12.));
#3663=CARTESIAN_POINT('',(4.76969600708473,-1.5,0.));
#3664=CARTESIAN_POINT('',(4.76969600708473,-1.5,0.));
#3665=CARTESIAN_POINT('',(6.,-1.5,12.));
#3666=CARTESIAN_POINT('',(3.,-1.5,12.));
#3667=CARTESIAN_POINT('',(6.,-1.5,0.));
#3668=CARTESIAN_POINT('',(6.,-1.5,12.));
#3669=CARTESIAN_POINT('',(3.,-1.5,0.));
#3670=CARTESIAN_POINT('Origin',(6.,1.5,12.));
#3671=CARTESIAN_POINT('',(6.,0.75,12.));
#3672=CARTESIAN_POINT('',(6.,0.75,0.));
#3673=CARTESIAN_POINT('Origin',(0.,0.,0.));
#3674=CARTESIAN_POINT('Origin',(0.,0.,12.));
#3675=CARTESIAN_POINT('Origin',(0.,0.,0.));
#3676=CARTESIAN_POINT('Origin',(0.,0.,12.));
#3677=CARTESIAN_POINT('',(-36.8837494704647,-82.095,12.));
#3678=CARTESIAN_POINT('',(36.8837494704646,-82.095,12.));
#3679=CARTESIAN_POINT('Origin',(-1.83697019872103E-14,-100.,12.));
#3680=CARTESIAN_POINT('',(39.7037362185807,-80.7688883808943,12.));
#3681=CARTESIAN_POINT('Origin',(0.,0.,12.));
#3682=CARTESIAN_POINT('',(15.8038475772934,-39.3730669589464,12.));
#3683=CARTESIAN_POINT('',(19.8038475772934,-46.3012701892219,12.));
#3684=CARTESIAN_POINT('',(26.1961524227066,-33.3730669589464,12.));
#3685=CARTESIAN_POINT('Origin',(21.,-36.3730669589464,12.));
#3686=CARTESIAN_POINT('',(50.0960410639939,-74.7688883808943,12.));
#3687=CARTESIAN_POINT('',(15.6961524227066,-15.1865334794732,12.));
#3688=CARTESIAN_POINT('',(52.6544807884511,-72.9897640282432,12.));
#3689=CARTESIAN_POINT('Origin',(0.,0.,12.));
#3690=CARTESIAN_POINT('',(89.5382302589158,-9.10523597175683,12.));
#3691=CARTESIAN_POINT('Origin',(86.6025403784438,-50.,12.));
#3692=CARTESIAN_POINT('',(89.7997772825746,-6.,12.));
#3693=CARTESIAN_POINT('Origin',(0.,0.,12.));
#3694=CARTESIAN_POINT('',(42.,-6.,12.));
#3695=CARTESIAN_POINT('',(50.,-6.,12.));
#3696=CARTESIAN_POINT('',(42.,6.,12.));
#3697=CARTESIAN_POINT('Origin',(42.,0.,12.));
#3698=CARTESIAN_POINT('',(89.7997772825746,6.,12.));
#3699=CARTESIAN_POINT('',(21.,6.,12.));
#3700=CARTESIAN_POINT('',(89.5382302589158,9.10523597175679,12.));
#3701=CARTESIAN_POINT('Origin',(0.,0.,12.));
#3702=CARTESIAN_POINT('',(52.6544807884512,72.9897640282432,12.));
#3703=CARTESIAN_POINT('Origin',(86.6025403784439,50.,12.));
#3704=CARTESIAN_POINT('',(50.0960410639939,74.7688883808943,12.));
#3705=CARTESIAN_POINT('Origin',(0.,0.,12.));
#3706=CARTESIAN_POINT('',(26.1961524227066,33.3730669589464,12.));
#3707=CARTESIAN_POINT('',(30.1961524227066,40.3012701892219,12.));
#3708=CARTESIAN_POINT('',(15.8038475772934,39.3730669589464,12.));
#3709=CARTESIAN_POINT('Origin',(21.,36.3730669589464,12.));
#3710=CARTESIAN_POINT('',(39.7037362185807,80.7688883808943,12.));
#3711=CARTESIAN_POINT('',(5.30384757729338,21.1865334794732,12.));
#3712=CARTESIAN_POINT('',(36.8837494704646,82.095,12.));
#3713=CARTESIAN_POINT('Origin',(0.,0.,12.));
#3714=CARTESIAN_POINT('',(-36.8837494704646,82.095,12.));
#3715=CARTESIAN_POINT('Origin',(6.12323399573677E-15,100.,12.));
#3716=CARTESIAN_POINT('',(-39.7037362185806,80.7688883808943,12.));
#3717=CARTESIAN_POINT('Origin',(0.,0.,12.));
#3718=CARTESIAN_POINT('',(-15.8038475772934,39.3730669589464,12.));
#3719=CARTESIAN_POINT('',(-19.8038475772934,46.3012701892219,12.));
#3720=CARTESIAN_POINT('',(-26.1961524227066,33.3730669589464,12.));
#3721=CARTESIAN_POINT('Origin',(-21.,36.3730669589464,12.));
#3722=CARTESIAN_POINT('',(-50.0960410639939,74.7688883808943,12.));
#3723=CARTESIAN_POINT('',(-15.6961524227066,15.1865334794732,12.));
#3724=CARTESIAN_POINT('',(-52.6544807884512,72.9897640282432,12.));
#3725=CARTESIAN_POINT('Origin',(0.,0.,12.));
#3726=CARTESIAN_POINT('',(-89.5382302589158,9.10523597175679,12.));
#3727=CARTESIAN_POINT('Origin',(-86.6025403784439,50.,12.));
#3728=CARTESIAN_POINT('',(-89.7997772825746,6.00000000000001,12.));
#3729=CARTESIAN_POINT('Origin',(0.,0.,12.));
#3730=CARTESIAN_POINT('',(-42.,6.00000000000001,12.));
#3731=CARTESIAN_POINT('',(-50.,6.00000000000001,12.));
#3732=CARTESIAN_POINT('',(-42.,-5.99999999999999,12.));
#3733=CARTESIAN_POINT('Origin',(-42.,5.14351655641888E-15,12.));
#3734=CARTESIAN_POINT('',(-89.7997772825746,-5.99999999999999,12.));
#3735=CARTESIAN_POINT('',(-21.,-6.,12.));
#3736=CARTESIAN_POINT('',(-89.5382302589158,-9.10523597175682,12.));
#3737=CARTESIAN_POINT('Origin',(0.,0.,12.));
#3738=CARTESIAN_POINT('',(-52.6544807884512,-72.9897640282432,12.));
#3739=CARTESIAN_POINT('Origin',(-86.6025403784438,-50.,12.));
#3740=CARTESIAN_POINT('',(-50.096041063994,-74.7688883808943,12.));
#3741=CARTESIAN_POINT('Origin',(0.,0.,12.));
#3742=CARTESIAN_POINT('',(-26.1961524227066,-33.3730669589464,12.));
#3743=CARTESIAN_POINT('',(-30.1961524227066,-40.3012701892219,12.));
#3744=CARTESIAN_POINT('',(-15.8038475772934,-39.3730669589464,12.));
#3745=CARTESIAN_POINT('Origin',(-21.,-36.3730669589464,12.));
#3746=CARTESIAN_POINT('',(-39.7037362185807,-80.7688883808943,12.));
#3747=CARTESIAN_POINT('',(-5.30384757729338,-21.1865334794732,12.));
#3748=CARTESIAN_POINT('Origin',(0.,0.,12.));
#3749=CARTESIAN_POINT('Origin',(-1.83697019872103E-14,-100.,6.));
#3750=CARTESIAN_POINT('',(36.8837494704646,-82.095,0.));
#3751=CARTESIAN_POINT('',(36.8837494704646,-82.095,6.));
#3752=CARTESIAN_POINT('',(-36.8837494704647,-82.095,0.));
#3753=CARTESIAN_POINT('',(-36.8837494704647,-82.095,6.));
#3754=CARTESIAN_POINT('Origin',(-1.83697019872103E-14,-100.,0.));
#3755=CARTESIAN_POINT('Origin',(-86.6025403784439,50.,6.));
#3756=CARTESIAN_POINT('',(-89.5382302589158,9.10523597175678,0.));
#3757=CARTESIAN_POINT('',(-89.5382302589158,9.10523597175678,6.));
#3758=CARTESIAN_POINT('',(-52.6544807884512,72.9897640282432,0.));
#3759=CARTESIAN_POINT('',(-52.6544807884512,72.9897640282432,6.));
#3760=CARTESIAN_POINT('Origin',(-86.6025403784439,50.,0.));
#3761=CARTESIAN_POINT('Origin',(86.6025403784439,50.,6.));
#3762=CARTESIAN_POINT('',(52.6544807884512,72.9897640282432,0.));
#3763=CARTESIAN_POINT('',(52.6544807884512,72.9897640282432,6.));
#3764=CARTESIAN_POINT('',(89.5382302589158,9.10523597175678,0.));
#3765=CARTESIAN_POINT('',(89.5382302589158,9.10523597175678,6.));
#3766=CARTESIAN_POINT('Origin',(86.6025403784439,50.,0.));
#3767=CARTESIAN_POINT('Origin',(6.12323399573677E-15,100.,6.));
#3768=CARTESIAN_POINT('',(-36.8837494704646,82.095,0.));
#3769=CARTESIAN_POINT('',(-36.8837494704646,82.095,6.));
#3770=CARTESIAN_POINT('',(36.8837494704646,82.095,0.));
#3771=CARTESIAN_POINT('',(36.8837494704646,82.095,6.));
#3772=CARTESIAN_POINT('Origin',(6.12323399573677E-15,100.,0.));
#3773=CARTESIAN_POINT('Origin',(-86.6025403784438,-50.,6.));
#3774=CARTESIAN_POINT('',(-52.6544807884512,-72.9897640282432,0.));
#3775=CARTESIAN_POINT('',(-52.6544807884512,-72.9897640282432,6.));
#3776=CARTESIAN_POINT('',(-89.5382302589158,-9.10523597175679,0.));
#3777=CARTESIAN_POINT('',(-89.5382302589158,-9.10523597175679,6.));
#3778=CARTESIAN_POINT('Origin',(-86.6025403784438,-50.,0.));
#3779=CARTESIAN_POINT('Origin',(86.6025403784438,-50.,6.));
#3780=CARTESIAN_POINT('',(52.6544807884511,-72.9897640282432,0.));
#3781=CARTESIAN_POINT('',(52.6544807884511,-72.9897640282432,6.));
#3782=CARTESIAN_POINT('',(89.5382302589158,-9.10523597175683,0.));
#3783=CARTESIAN_POINT('Origin',(86.6025403784438,-50.,0.));
#3784=CARTESIAN_POINT('',(89.5382302589158,-9.10523597175683,6.));
#3785=CARTESIAN_POINT('Origin',(0.,0.,0.));
#3786=CARTESIAN_POINT('',(-39.7037362185807,-80.7688883808943,0.));
#3787=CARTESIAN_POINT('',(-39.7037362185807,-80.7688883808943,0.));
#3788=CARTESIAN_POINT('Origin',(0.,0.,0.));
#3789=CARTESIAN_POINT('Origin',(0.,0.,0.));
#3790=CARTESIAN_POINT('',(39.7037362185807,-80.7688883808943,0.));
#3791=CARTESIAN_POINT('Origin',(0.,0.,0.));
#3792=CARTESIAN_POINT('',(39.7037362185807,-80.7688883808943,0.));
#3793=CARTESIAN_POINT('Origin',(0.,0.,0.));
#3794=CARTESIAN_POINT('',(-50.0960410639939,74.7688883808943,0.));
#3795=CARTESIAN_POINT('',(-50.0960410639939,74.7688883808943,0.));
#3796=CARTESIAN_POINT('Origin',(0.,0.,0.));
#3797=CARTESIAN_POINT('Origin',(0.,0.,0.));
#3798=CARTESIAN_POINT('',(89.7997772825746,6.,0.));
#3799=CARTESIAN_POINT('',(89.7997772825746,6.,0.));
#3800=CARTESIAN_POINT('Origin',(0.,0.,0.));
#3801=CARTESIAN_POINT('Origin',(0.,0.,0.));
#3802=CARTESIAN_POINT('',(39.7037362185807,80.7688883808943,0.));
#3803=CARTESIAN_POINT('',(39.7037362185807,80.7688883808943,0.));
#3804=CARTESIAN_POINT('Origin',(0.,0.,0.));
#3805=CARTESIAN_POINT('Origin',(0.,0.,0.));
#3806=CARTESIAN_POINT('',(-89.7997772825746,-5.99999999999999,0.));
#3807=CARTESIAN_POINT('',(-89.7997772825746,-5.99999999999999,0.));
#3808=CARTESIAN_POINT('Origin',(0.,0.,0.));
#3809=CARTESIAN_POINT('Origin',(0.,0.,0.));
#3810=CARTESIAN_POINT('',(-15.8038475772934,-39.3730669589464,0.));
#3811=CARTESIAN_POINT('',(-5.30384757729338,-21.1865334794732,0.));
#3812=CARTESIAN_POINT('',(-26.1961524227066,-33.3730669589464,0.));
#3813=CARTESIAN_POINT('Origin',(-21.,-36.3730669589464,0.));
#3814=CARTESIAN_POINT('',(-50.096041063994,-74.7688883808943,0.));
#3815=CARTESIAN_POINT('',(-30.1961524227066,-40.3012701892219,0.));
#3816=CARTESIAN_POINT('Origin',(0.,0.,0.));
#3817=CARTESIAN_POINT('',(-42.,-5.99999999999999,0.));
#3818=CARTESIAN_POINT('',(-21.,-6.,0.));
#3819=CARTESIAN_POINT('',(-42.,6.00000000000001,0.));
#3820=CARTESIAN_POINT('Origin',(-42.,5.14351655641888E-15,0.));
#3821=CARTESIAN_POINT('',(-89.7997772825746,6.00000000000001,0.));
#3822=CARTESIAN_POINT('',(-50.,6.00000000000001,0.));
#3823=CARTESIAN_POINT('Origin',(0.,0.,0.));
#3824=CARTESIAN_POINT('',(-26.1961524227066,33.3730669589464,0.));
#3825=CARTESIAN_POINT('',(-15.6961524227066,15.1865334794732,0.));
#3826=CARTESIAN_POINT('',(-15.8038475772934,39.3730669589464,0.));
#3827=CARTESIAN_POINT('Origin',(-21.,36.3730669589464,0.));
#3828=CARTESIAN_POINT('',(-39.7037362185806,80.7688883808943,0.));
#3829=CARTESIAN_POINT('',(-19.8038475772934,46.3012701892219,0.));
#3830=CARTESIAN_POINT('Origin',(0.,0.,0.));
#3831=CARTESIAN_POINT('',(15.8038475772934,39.3730669589464,0.));
#3832=CARTESIAN_POINT('',(5.30384757729338,21.1865334794732,1.11022302462516E-15));
#3833=CARTESIAN_POINT('',(26.1961524227066,33.3730669589464,0.));
#3834=CARTESIAN_POINT('Origin',(21.,36.3730669589464,0.));
#3835=CARTESIAN_POINT('',(50.0960410639939,74.7688883808943,0.));
#3836=CARTESIAN_POINT('',(30.1961524227066,40.3012701892219,0.));
#3837=CARTESIAN_POINT('Origin',(0.,0.,0.));
#3838=CARTESIAN_POINT('',(42.,6.,0.));
#3839=CARTESIAN_POINT('',(21.,6.,0.));
#3840=CARTESIAN_POINT('',(42.,-6.,0.));
#3841=CARTESIAN_POINT('Origin',(42.,0.,0.));
#3842=CARTESIAN_POINT('',(89.7997772825746,-6.,0.));
#3843=CARTESIAN_POINT('',(50.,-6.,0.));
#3844=CARTESIAN_POINT('Origin',(0.,0.,0.));
#3845=CARTESIAN_POINT('',(50.0960410639939,-74.7688883808943,0.));
#3846=CARTESIAN_POINT('Origin',(0.,0.,0.));
#3847=CARTESIAN_POINT('',(26.1961524227066,-33.3730669589464,0.));
#3848=CARTESIAN_POINT('',(15.6961524227066,-15.1865334794732,0.));
#3849=CARTESIAN_POINT('',(15.8038475772934,-39.3730669589464,0.));
#3850=CARTESIAN_POINT('Origin',(21.,-36.3730669589464,0.));
#3851=CARTESIAN_POINT('',(19.8038475772934,-46.3012701892219,1.11022302462516E-15));
#3852=CARTESIAN_POINT('Origin',(0.,0.,0.));
#3853=CARTESIAN_POINT('',(89.7997772825746,-6.,0.));
#3854=CARTESIAN_POINT('Origin',(0.,0.,0.));
#3855=CARTESIAN_POINT('',(50.0960410639939,-74.7688883808943,0.));
#3856=CARTESIAN_POINT('Origin',(44.8038475772934,-89.6025403784439,12.));
#3857=CARTESIAN_POINT('',(15.8038475772934,-39.3730669589464,12.));
#3858=CARTESIAN_POINT('Origin',(26.1961524227066,-33.3730669589464,12.));
#3859=CARTESIAN_POINT('',(26.1961524227066,-33.3730669589464,12.));
#3860=CARTESIAN_POINT('Origin',(21.,-36.3730669589464,12.));
#3861=CARTESIAN_POINT('Origin',(-55.1961524227066,-83.6025403784438,12.));
#3862=CARTESIAN_POINT('',(-50.096041063994,-74.7688883808943,0.));
#3863=CARTESIAN_POINT('',(-26.1961524227066,-33.3730669589464,12.));
#3864=CARTESIAN_POINT('Origin',(-15.8038475772934,-39.3730669589464,12.));
#3865=CARTESIAN_POINT('',(-15.8038475772934,-39.3730669589464,12.));
#3866=CARTESIAN_POINT('Origin',(-21.,-36.3730669589464,12.));
#3867=CARTESIAN_POINT('Origin',(-100.,6.00000000000001,12.));
#3868=CARTESIAN_POINT('',(-89.7997772825746,6.00000000000001,0.));
#3869=CARTESIAN_POINT('',(-42.,6.00000000000001,12.));
#3870=CARTESIAN_POINT('Origin',(-42.,-5.99999999999999,12.));
#3871=CARTESIAN_POINT('',(-42.,-5.99999999999999,12.));
#3872=CARTESIAN_POINT('Origin',(-42.,5.14351655641888E-15,12.));
#3873=CARTESIAN_POINT('Origin',(0.,0.,0.));
#3874=CARTESIAN_POINT('Origin',(0.,0.,0.));
#3875=CARTESIAN_POINT('Origin',(-44.8038475772934,89.6025403784439,12.));
#3876=CARTESIAN_POINT('',(-39.7037362185806,80.7688883808943,0.));
#3877=CARTESIAN_POINT('',(-15.8038475772934,39.3730669589464,12.));
#3878=CARTESIAN_POINT('Origin',(-26.1961524227066,33.3730669589464,12.));
#3879=CARTESIAN_POINT('',(-26.1961524227066,33.3730669589464,12.));
#3880=CARTESIAN_POINT('Origin',(-21.,36.3730669589464,12.));
#3881=CARTESIAN_POINT('Origin',(55.1961524227066,83.6025403784438,12.));
#3882=CARTESIAN_POINT('',(50.0960410639939,74.7688883808943,0.));
#3883=CARTESIAN_POINT('',(26.1961524227066,33.3730669589464,12.));
#3884=CARTESIAN_POINT('Origin',(15.8038475772934,39.3730669589464,12.));
#3885=CARTESIAN_POINT('',(15.8038475772934,39.3730669589464,12.));
#3886=CARTESIAN_POINT('Origin',(21.,36.3730669589464,12.));
#3887=CARTESIAN_POINT('Origin',(0.,0.,0.));
#3888=CARTESIAN_POINT('Origin',(0.,0.,0.));
#3889=CARTESIAN_POINT('Origin',(100.,-6.,12.));
#3890=CARTESIAN_POINT('',(42.,-6.,12.));
#3891=CARTESIAN_POINT('Origin',(42.,6.,12.));
#3892=CARTESIAN_POINT('',(42.,6.,12.));
#3893=CARTESIAN_POINT('Origin',(42.,0.,12.));
#4127=UNCERTAINTY_MEASURE_WITH_UNIT(LENGTH_MEASURE(0.01),#4150,
'DISTANCE_ACCURACY_VALUE',
'Maximum model space distance between geometric entities at asserted c
onnectivities');
#4136=UNCERTAINTY_MEASURE_WITH_UNIT(LENGTH_MEASURE(0.01),#4150,
'DISTANCE_ACCURACY_VALUE',
'Maximum model space distance between geometric entities at asserted c
onnectivities');
#4140=(
GEOMETRIC_REPRESENTATION_CONTEXT(3)
GLOBAL_UNCERTAINTY_ASSIGNED_CONTEXT((#4127))
GLOBAL_UNIT_ASSIGNED_CONTEXT((#4150,#4152,#4153))
REPRESENTATION_CONTEXT('','3D')
);
#4149=(
GEOMETRIC_REPRESENTATION_CONTEXT(3)
GLOBAL_UNCERTAINTY_ASSIGNED_CONTEXT((#4136))
GLOBAL_UNIT_ASSIGNED_CONTEXT((#4150,#4152,#4153))
REPRESENTATION_CONTEXT('','3D')
);
#4150=(
LENGTH_UNIT()
NAMED_UNIT(*)
SI_UNIT(.MILLI.,.METRE.)
);
#4152=(
NAMED_UNIT(*)
PLANE_ANGLE_UNIT()
SI_UNIT($,.RADIAN.)
);
#4153=(
NAMED_UNIT(*)
SI_UNIT($,.STERADIAN.)
SOLID_ANGLE_UNIT()
);
#4157=SHAPE_DEFINITION_REPRESENTATION(#4169,#4198);
#4169=PRODUCT_DEFINITION_SHAPE('',$,#4211);
#4198=SHAPE_REPRESENTATION('',(#2502),#4140);
#4207=PRODUCT_DEFINITION_CONTEXT('part definition',#4245,'design');
#4211=PRODUCT_DEFINITION('Indexing starwheel','Indexing starwheel',#4223,
#4207);
#4223=PRODUCT_DEFINITION_FORMATION('',$,#4250);
#4245=APPLICATION_CONTEXT(
'Core Data for Automotive Mechanical Design Process');
#4246=PRODUCT_CONTEXT('part definition',#4245,'mechanical');
#4250=PRODUCT('Indexing starwheel','Indexing starwheel',$,(#4246));
#4262=PRESENTATION_STYLE_ASSIGNMENT((#4272));
#4272=SURFACE_STYLE_USAGE(.BOTH.,#4282);
#4282=SURFACE_SIDE_STYLE('',(#4292));
#4292=SURFACE_STYLE_FILL_AREA(#4302);
#4302=FILL_AREA_STYLE('Sky blue',(#4312));
#4312=FILL_AREA_STYLE_COLOUR('Sky blue',#4322);
#4322=COLOUR_RGB('Sky blue',0.317647058823529,0.686274509803922,0.890196078431372);
ENDSEC;
END-ISO-10303-21;
